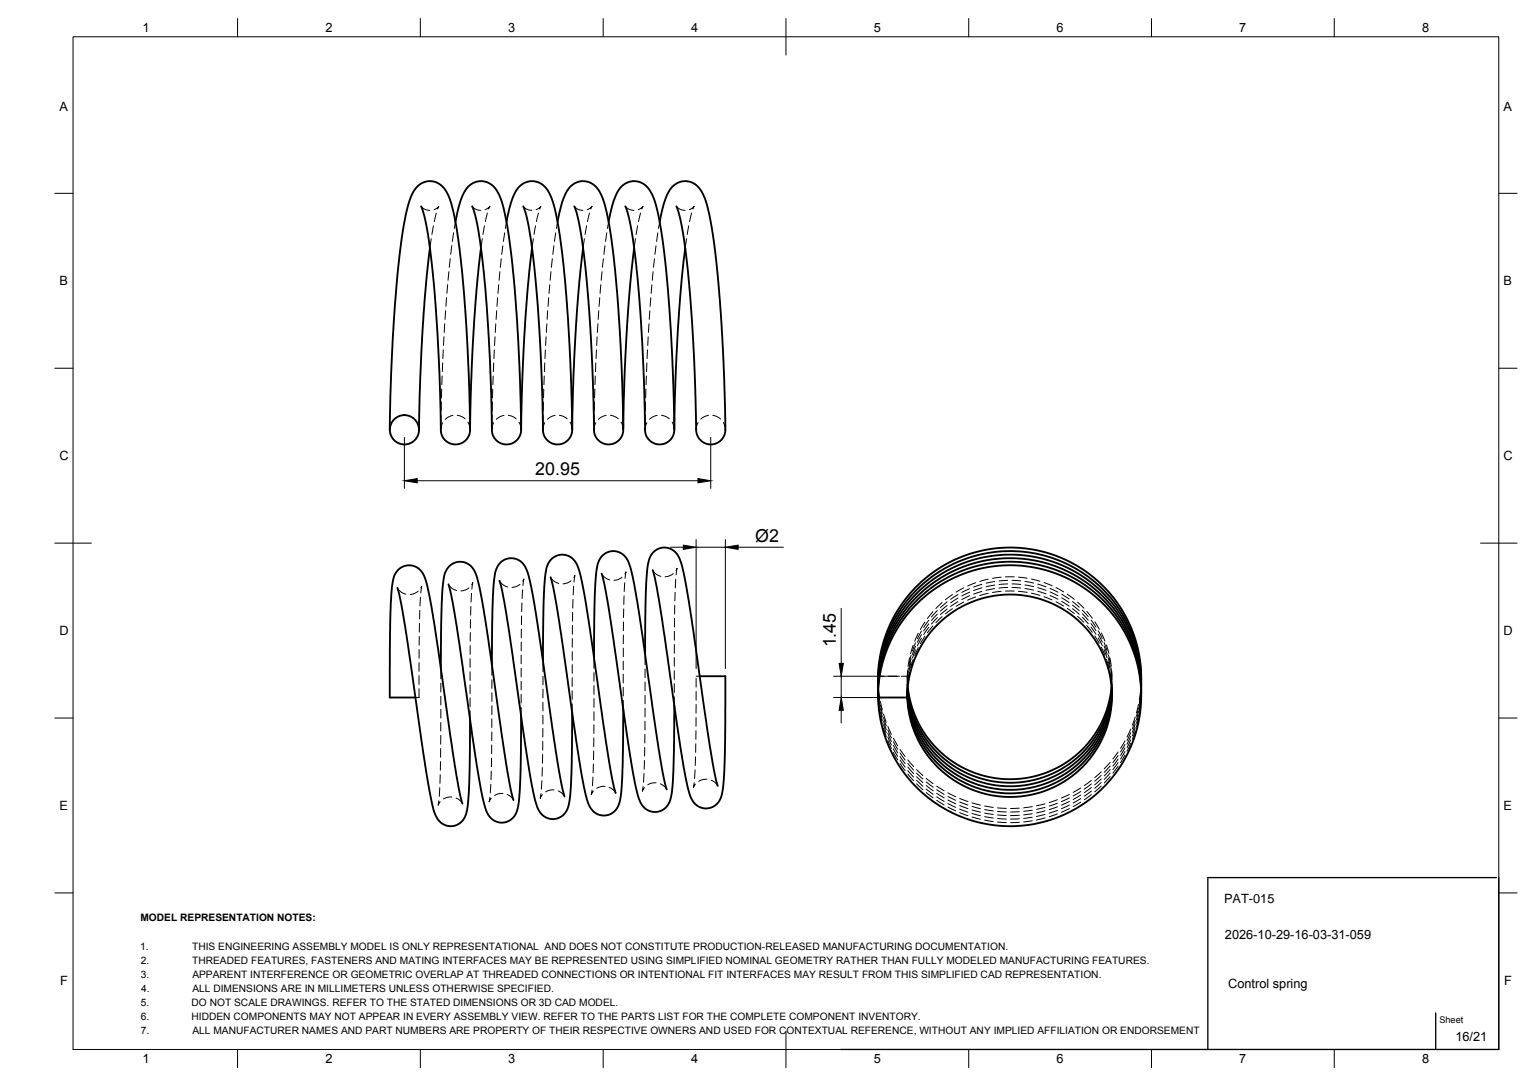
ISO-10303-21;
HEADER;
/* Generated by software containing ST-Developer
 * from STEP Tools, Inc. (www.steptools.com) 
 */

FILE_DESCRIPTION(
/* description */ ('PAT-015'),
/* implementation_level */ '2;1');

FILE_NAME(
/* name */ 'Control spring.step',
/* time_stamp */ '2026-10-29T16:03:43-07:00',
/* author */ (''),
/* organization */ (''),
/* preprocessor_version */ 'ST-DEVELOPER v20.2',
/* originating_system */ 'Autodesk Translation Framework v15.17.0.0',
/* authorisation */ '');

FILE_SCHEMA (('AUTOMOTIVE_DESIGN { 1 0 10303 214 3 1 1 }'));
ENDSEC;

DATA;
#10=MECHANICAL_DESIGN_GEOMETRIC_PRESENTATION_REPRESENTATION('',(#244),#10266);
#167=B_SPLINE_SURFACE_WITH_KNOTS('',3,3,((#8962,#8963,#8964,#8965,#8966,
#8967,#8968,#8969,#8970,#8971,#8972,#8973,#8974,#8975,#8976,#8977,#8978,
#8979,#8980,#8981,#8982,#8983,#8984,#8985,#8986,#8987,#8988,#8989,#8990,
#8991,#8992,#8993,#8994,#8995,#8996,#8997,#8998,#8999,#9000,#9001,#9002,
#9003,#9004,#9005,#9006,#9007,#9008,#9009,#9010,#9011,#9012,#9013,#9014,
#9015,#9016,#9017,#9018,#9019,#9020,#9021,#9022,#9023,#9024,#9025,#9026,
#9027,#9028,#9029,#9030,#9031,#9032),(#9033,#9034,#9035,#9036,#9037,#9038,
#9039,#9040,#9041,#9042,#9043,#9044,#9045,#9046,#9047,#9048,#9049,#9050,
#9051,#9052,#9053,#9054,#9055,#9056,#9057,#9058,#9059,#9060,#9061,#9062,
#9063,#9064,#9065,#9066,#9067,#9068,#9069,#9070,#9071,#9072,#9073,#9074,
#9075,#9076,#9077,#9078,#9079,#9080,#9081,#9082,#9083,#9084,#9085,#9086,
#9087,#9088,#9089,#9090,#9091,#9092,#9093,#9094,#9095,#9096,#9097,#9098,
#9099,#9100,#9101,#9102,#9103),(#9104,#9105,#9106,#9107,#9108,#9109,#9110,
#9111,#9112,#9113,#9114,#9115,#9116,#9117,#9118,#9119,#9120,#9121,#9122,
#9123,#9124,#9125,#9126,#9127,#9128,#9129,#9130,#9131,#9132,#9133,#9134,
#9135,#9136,#9137,#9138,#9139,#9140,#9141,#9142,#9143,#9144,#9145,#9146,
#9147,#9148,#9149,#9150,#9151,#9152,#9153,#9154,#9155,#9156,#9157,#9158,
#9159,#9160,#9161,#9162,#9163,#9164,#9165,#9166,#9167,#9168,#9169,#9170,
#9171,#9172,#9173,#9174),(#9175,#9176,#9177,#9178,#9179,#9180,#9181,#9182,
#9183,#9184,#9185,#9186,#9187,#9188,#9189,#9190,#9191,#9192,#9193,#9194,
#9195,#9196,#9197,#9198,#9199,#9200,#9201,#9202,#9203,#9204,#9205,#9206,
#9207,#9208,#9209,#9210,#9211,#9212,#9213,#9214,#9215,#9216,#9217,#9218,
#9219,#9220,#9221,#9222,#9223,#9224,#9225,#9226,#9227,#9228,#9229,#9230,
#9231,#9232,#9233,#9234,#9235,#9236,#9237,#9238,#9239,#9240,#9241,#9242,
#9243,#9244,#9245),(#9246,#9247,#9248,#9249,#9250,#9251,#9252,#9253,#9254,
#9255,#9256,#9257,#9258,#9259,#9260,#9261,#9262,#9263,#9264,#9265,#9266,
#9267,#9268,#9269,#9270,#9271,#9272,#9273,#9274,#9275,#9276,#9277,#9278,
#9279,#9280,#9281,#9282,#9283,#9284,#9285,#9286,#9287,#9288,#9289,#9290,
#9291,#9292,#9293,#9294,#9295,#9296,#9297,#9298,#9299,#9300,#9301,#9302,
#9303,#9304,#9305,#9306,#9307,#9308,#9309,#9310,#9311,#9312,#9313,#9314,
#9315,#9316),(#9317,#9318,#9319,#9320,#9321,#9322,#9323,#9324,#9325,#9326,
#9327,#9328,#9329,#9330,#9331,#9332,#9333,#9334,#9335,#9336,#9337,#9338,
#9339,#9340,#9341,#9342,#9343,#9344,#9345,#9346,#9347,#9348,#9349,#9350,
#9351,#9352,#9353,#9354,#9355,#9356,#9357,#9358,#9359,#9360,#9361,#9362,
#9363,#9364,#9365,#9366,#9367,#9368,#9369,#9370,#9371,#9372,#9373,#9374,
#9375,#9376,#9377,#9378,#9379,#9380,#9381,#9382,#9383,#9384,#9385,#9386,
#9387),(#9388,#9389,#9390,#9391,#9392,#9393,#9394,#9395,#9396,#9397,#9398,
#9399,#9400,#9401,#9402,#9403,#9404,#9405,#9406,#9407,#9408,#9409,#9410,
#9411,#9412,#9413,#9414,#9415,#9416,#9417,#9418,#9419,#9420,#9421,#9422,
#9423,#9424,#9425,#9426,#9427,#9428,#9429,#9430,#9431,#9432,#9433,#9434,
#9435,#9436,#9437,#9438,#9439,#9440,#9441,#9442,#9443,#9444,#9445,#9446,
#9447,#9448,#9449,#9450,#9451,#9452,#9453,#9454,#9455,#9456,#9457,#9458),
(#9459,#9460,#9461,#9462,#9463,#9464,#9465,#9466,#9467,#9468,#9469,#9470,
#9471,#9472,#9473,#9474,#9475,#9476,#9477,#9478,#9479,#9480,#9481,#9482,
#9483,#9484,#9485,#9486,#9487,#9488,#9489,#9490,#9491,#9492,#9493,#9494,
#9495,#9496,#9497,#9498,#9499,#9500,#9501,#9502,#9503,#9504,#9505,#9506,
#9507,#9508,#9509,#9510,#9511,#9512,#9513,#9514,#9515,#9516,#9517,#9518,
#9519,#9520,#9521,#9522,#9523,#9524,#9525,#9526,#9527,#9528,#9529),(#9530,
#9531,#9532,#9533,#9534,#9535,#9536,#9537,#9538,#9539,#9540,#9541,#9542,
#9543,#9544,#9545,#9546,#9547,#9548,#9549,#9550,#9551,#9552,#9553,#9554,
#9555,#9556,#9557,#9558,#9559,#9560,#9561,#9562,#9563,#9564,#9565,#9566,
#9567,#9568,#9569,#9570,#9571,#9572,#9573,#9574,#9575,#9576,#9577,#9578,
#9579,#9580,#9581,#9582,#9583,#9584,#9585,#9586,#9587,#9588,#9589,#9590,
#9591,#9592,#9593,#9594,#9595,#9596,#9597,#9598,#9599,#9600),(#9601,#9602,
#9603,#9604,#9605,#9606,#9607,#9608,#9609,#9610,#9611,#9612,#9613,#9614,
#9615,#9616,#9617,#9618,#9619,#9620,#9621,#9622,#9623,#9624,#9625,#9626,
#9627,#9628,#9629,#9630,#9631,#9632,#9633,#9634,#9635,#9636,#9637,#9638,
#9639,#9640,#9641,#9642,#9643,#9644,#9645,#9646,#9647,#9648,#9649,#9650,
#9651,#9652,#9653,#9654,#9655,#9656,#9657,#9658,#9659,#9660,#9661,#9662,
#9663,#9664,#9665,#9666,#9667,#9668,#9669,#9670,#9671)),.UNSPECIFIED.,.T.,
 .F.,.F.,(4,1,1,1,1,1,1,4),(4,1,1,1,1,1,1,1,1,1,1,1,1,1,1,1,1,1,1,1,1,1,
1,1,1,1,1,1,1,1,1,1,1,1,1,1,1,1,1,1,1,1,1,1,1,1,1,1,1,1,1,1,1,1,1,1,1,1,
1,1,1,1,1,1,1,1,1,1,4),(-3.14159265358979,-2.24399475256414,-1.34639685153848,
-0.448798950512828,0.448798950512828,1.34639685153848,2.24399475256414,
3.14159265358979),(0.,0.0178571428571429,0.0357142857142857,0.0535714285714286,
0.0714285714285714,0.0892857142857143,0.107142857142857,0.125,0.142857142857143,
0.150793650793651,0.158730158730159,0.174603174603175,0.19047619047619,
0.202380952380952,0.214285714285714,0.226190476190476,0.238095238095238,
0.25,0.261904761904762,0.267857142857143,0.273809523809524,0.285714285714286,
0.297619047619048,0.30952380952381,0.321428571428571,0.333333333333333,
0.349206349206349,0.365079365079365,0.380952380952381,0.396825396825397,
0.412698412698413,0.428571428571429,0.446428571428571,0.464285714285714,
0.476190476190476,0.488095238095238,0.5,0.517857142857143,0.535714285714286,
0.553571428571429,0.571428571428571,0.589285714285714,0.607142857142857,
0.625,0.642857142857143,0.660714285714286,0.678571428571428,0.696428571428571,
0.714285714285714,0.726190476190476,0.738095238095238,0.75,0.761904761904762,
0.773809523809524,0.785714285714286,0.797619047619047,0.809523809523809,
0.821428571428571,0.833333333333333,0.845238095238095,0.857142857142857,
0.875,0.892857142857143,0.910714285714286,0.928571428571429,0.946428571428571,
0.964285714285714,0.982142857142857,1.),.UNSPECIFIED.);
#196=SHAPE_REPRESENTATION_RELATIONSHIP('SRR','None',#10367,#219);
#219=ADVANCED_BREP_SHAPE_REPRESENTATION('',(#269),#10255);
#244=STYLED_ITEM('',(#10547),#269);
#269=MANIFOLD_SOLID_BREP('Body1',#4703);
#513=PLANE('',#5380);
#514=PLANE('',#5381);
#767=FACE_OUTER_BOUND('',#1164,.T.);
#768=FACE_OUTER_BOUND('',#1165,.T.);
#769=FACE_OUTER_BOUND('',#1166,.T.);
#1164=EDGE_LOOP('',(#3963,#3964,#3965,#3966));
#1165=EDGE_LOOP('',(#3967));
#1166=EDGE_LOOP('',(#3968));
#1319=B_SPLINE_CURVE_WITH_KNOTS('',3,(#9675,#9676,#9677,#9678,#9679,#9680,
#9681,#9682,#9683,#9684,#9685,#9686,#9687,#9688,#9689,#9690,#9691,#9692,
#9693,#9694,#9695,#9696,#9697,#9698,#9699,#9700,#9701,#9702,#9703,#9704,
#9705,#9706,#9707,#9708,#9709,#9710,#9711,#9712,#9713,#9714,#9715,#9716,
#9717,#9718,#9719,#9720,#9721,#9722,#9723,#9724,#9725,#9726,#9727,#9728,
#9729,#9730,#9731,#9732,#9733,#9734,#9735,#9736,#9737,#9738,#9739,#9740,
#9741,#9742,#9743,#9744,#9745),.UNSPECIFIED.,.F.,.F.,(4,1,1,1,1,1,1,1,1,
1,1,1,1,1,1,1,1,1,1,1,1,1,1,1,1,1,1,1,1,1,1,1,1,1,1,1,1,1,1,1,1,1,1,1,1,
1,1,1,1,1,1,1,1,1,1,1,1,1,1,1,1,1,1,1,1,1,1,1,4),(0.,0.0178571428571429,
0.0357142857142857,0.0535714285714286,0.0714285714285714,0.0892857142857143,
0.107142857142857,0.125,0.142857142857143,0.150793650793651,0.158730158730159,
0.174603174603175,0.19047619047619,0.202380952380952,0.214285714285714,
0.226190476190476,0.238095238095238,0.25,0.261904761904762,0.267857142857143,
0.273809523809524,0.285714285714286,0.297619047619048,0.30952380952381,
0.321428571428571,0.333333333333333,0.349206349206349,0.365079365079365,
0.380952380952381,0.396825396825397,0.412698412698413,0.428571428571429,
0.446428571428571,0.464285714285714,0.476190476190476,0.488095238095238,
0.5,0.517857142857143,0.535714285714286,0.553571428571429,0.571428571428571,
0.589285714285714,0.607142857142857,0.625,0.642857142857143,0.660714285714286,
0.678571428571428,0.696428571428571,0.714285714285714,0.726190476190476,
0.738095238095238,0.75,0.761904761904762,0.773809523809524,0.785714285714286,
0.797619047619047,0.809523809523809,0.821428571428571,0.833333333333333,
0.845238095238095,0.857142857142857,0.875,0.892857142857143,0.910714285714286,
0.928571428571429,0.946428571428571,0.964285714285714,0.982142857142857,
1.),.UNSPECIFIED.);
#2067=CIRCLE('',#5378,0.1);
#2068=CIRCLE('',#5379,0.1);
#2401=VERTEX_POINT('',#9672);
#2402=VERTEX_POINT('',#9674);
#2937=EDGE_CURVE('',#2401,#2401,#2067,.T.);
#2938=EDGE_CURVE('',#2401,#2402,#1319,.T.);
#2939=EDGE_CURVE('',#2402,#2402,#2068,.T.);
#3963=ORIENTED_EDGE('',*,*,#2937,.T.);
#3964=ORIENTED_EDGE('',*,*,#2938,.T.);
#3965=ORIENTED_EDGE('',*,*,#2939,.F.);
#3966=ORIENTED_EDGE('',*,*,#2938,.F.);
#3967=ORIENTED_EDGE('',*,*,#2939,.T.);
#3968=ORIENTED_EDGE('',*,*,#2937,.F.);
#4602=ADVANCED_FACE('',(#767),#167,.T.);
#4603=ADVANCED_FACE('',(#768),#513,.T.);
#4604=ADVANCED_FACE('',(#769),#514,.F.);
#4703=CLOSED_SHELL('',(#4602,#4603,#4604));
#5377=AXIS2_PLACEMENT_3D('',#8961,#6549,#6550);
#5378=AXIS2_PLACEMENT_3D('',#9673,#6551,#6552);
#5379=AXIS2_PLACEMENT_3D('',#9746,#6553,#6554);
#5380=AXIS2_PLACEMENT_3D('',#9747,#6555,#6556);
#5381=AXIS2_PLACEMENT_3D('',#9748,#6557,#6558);
#6549=DIRECTION('axis',(0.,0.,1.));
#6550=DIRECTION('refdir',(1.,0.,0.));
#6551=DIRECTION('center_axis',(-0.000134591856444243,0.997598919682403,
0.0692558830247305));
#6552=DIRECTION('ref_axis',(9.34371278597603E-6,-0.0692558823944232,0.997598928761687));
#6553=DIRECTION('center_axis',(0.000134591670588553,0.997598919668532,0.0692558832248945));
#6554=DIRECTION('ref_axis',(-0.499431472094232,0.0600671278230296,-0.864268560597272));
#6555=DIRECTION('center_axis',(0.000134591670588553,0.997598919668532,0.0692558832248945));
#6556=DIRECTION('ref_axis',(-0.499431472094232,0.0600671278230296,-0.864268560597272));
#6557=DIRECTION('center_axis',(-0.000134591856444243,0.997598919682403,
0.0692558830247305));
#6558=DIRECTION('ref_axis',(9.34371278597603E-6,-0.0692558823944232,0.997598928761687));
#8961=CARTESIAN_POINT('',(0.,0.,0.));
#8962=CARTESIAN_POINT('Ctrl Pts',(0.799999065628721,0.00692558823944229,
5.30024010712383));
#8963=CARTESIAN_POINT('Ctrl Pts',(0.799974755250737,0.187114846749742,5.31274930893178));
#8964=CARTESIAN_POINT('Ctrl Pts',(0.674578200671659,0.546127076651831,5.33781512365923));
#8965=CARTESIAN_POINT('Ctrl Pts',(0.187998995393781,0.852903359039399,5.37564381521248));
#8966=CARTESIAN_POINT('Ctrl Pts',(-0.386721866921525,0.788448388841122,
5.41368605209984));
#8967=CARTESIAN_POINT('Ctrl Pts',(-0.7983994419892,0.377627224111744,5.45194644400096));
#8968=CARTESIAN_POINT('Ctrl Pts',(-0.864375113399524,-0.203617876612744,
5.49042055747836));
#8969=CARTESIAN_POINT('Ctrl Pts',(-0.552019639313923,-0.701812288635587,
5.52910737914477));
#8970=CARTESIAN_POINT('Ctrl Pts',(0.00615426428515267,-0.897757418326962,
5.56800374230524));
#8971=CARTESIAN_POINT('Ctrl Pts',(0.463089276607972,-0.737891299975203,
5.59986549204054));
#8972=CARTESIAN_POINT('Ctrl Pts',(0.706662565433678,-0.474149107376678,
5.62457829573124));
#8973=CARTESIAN_POINT('Ctrl Pts',(0.854347338563578,-0.169471123140589,
5.6478904398873));
#8974=CARTESIAN_POINT('Ctrl Pts',(0.854381411403854,0.269671075667267,5.67712918390586));
#8975=CARTESIAN_POINT('Ctrl Pts',(0.581578462406747,0.670744438556907,5.70943359497258));
#8976=CARTESIAN_POINT('Ctrl Pts',(0.189982000930166,0.858805851522918,5.73891161848027));
#8977=CARTESIAN_POINT('Ctrl Pts',(-0.201854620920769,0.859148371452269,
5.76552549972421));
#8978=CARTESIAN_POINT('Ctrl Pts',(-0.556170302204947,0.688486751453872,
5.79222147180784));
#8979=CARTESIAN_POINT('Ctrl Pts',(-0.802120584542054,0.380288702719923,
5.81899788702529));
#8980=CARTESIAN_POINT('Ctrl Pts',(-0.890321102734134,-0.0053444036833259,
5.84585301727138));
#8981=CARTESIAN_POINT('Ctrl Pts',(-0.816781798992104,-0.327577127496462,
5.86829638740099));
#8982=CARTESIAN_POINT('Ctrl Pts',(-0.678277859648778,-0.547664335405585,
5.88628859994389));
#8983=CARTESIAN_POINT('Ctrl Pts',(-0.494316135451619,-0.731945478665225,
5.90430550175064));
#8984=CARTESIAN_POINT('Ctrl Pts',(-0.194941007989142,-0.876310026230692,
5.92687230420244));
#8985=CARTESIAN_POINT('Ctrl Pts',(0.204945568353256,-0.876409485122255,
5.95402353339188));
#8986=CARTESIAN_POINT('Ctrl Pts',(0.566325487118899,-0.702556101088839,
5.98124373289334));
#8987=CARTESIAN_POINT('Ctrl Pts',(0.816751045229916,-0.388463305588866,
6.00853075028047));
#8988=CARTESIAN_POINT('Ctrl Pts',(0.917174982875959,0.0480250206861584,
6.03892142694837));
#8989=CARTESIAN_POINT('Ctrl Pts',(0.768829350780382,0.528866010776267,6.07244001895545));
#8990=CARTESIAN_POINT('Ctrl Pts',(0.338627495917749,0.872873034891815,6.10911095186911));
#8991=CARTESIAN_POINT('Ctrl Pts',(-0.212178222814091,0.914151313349766,
6.14588130840082));
#8992=CARTESIAN_POINT('Ctrl Pts',(-0.691759933067223,0.637451614256161,
6.18274515756461));
#8993=CARTESIAN_POINT('Ctrl Pts',(-0.932934482256533,0.137697594997002,
6.21969639210087));
#8994=CARTESIAN_POINT('Ctrl Pts',(-0.84730393945114,-0.435496308403701,
6.25827178793966));
#8995=CARTESIAN_POINT('Ctrl Pts',(-0.415273257958933,-0.868240176171726,
6.29847623644814));
#8996=CARTESIAN_POINT('Ctrl Pts',(0.146189896678077,-0.930950222024402,
6.33566388079779));
#8997=CARTESIAN_POINT('Ctrl Pts',(0.578787425776111,-0.722091726547751,
6.36825221458814));
#8998=CARTESIAN_POINT('Ctrl Pts',(0.835229259505866,-0.400278931762148,
6.3962159259868));
#8999=CARTESIAN_POINT('Ctrl Pts',(0.943177486850013,0.0688606453452641,
6.42887288667825));
#9000=CARTESIAN_POINT('Ctrl Pts',(0.756462512495389,0.604750444420971,6.46623690685835));
#9001=CARTESIAN_POINT('Ctrl Pts',(0.214509054547464,0.945343920852135,6.50831791566041));
#9002=CARTESIAN_POINT('Ctrl Pts',(-0.421585054233784,0.873670673138226,
6.55043539297339));
#9003=CARTESIAN_POINT('Ctrl Pts',(-0.874725713994987,0.420703846750279,
6.59257924943873));
#9004=CARTESIAN_POINT('Ctrl Pts',(-0.946491736933492,-0.216206220818672,
6.63473932973225));
#9005=CARTESIAN_POINT('Ctrl Pts',(-0.605472064685913,-0.758979181442101,
6.67690544450194));
#9006=CARTESIAN_POINT('Ctrl Pts',(-0.000509641250504898,-0.970641038681315,
6.71906739492544));
#9007=CARTESIAN_POINT('Ctrl Pts',(0.604236817182525,-0.758999928674301,
6.76121498571335));
#9008=CARTESIAN_POINT('Ctrl Pts',(0.944676427167983,-0.216670516455945,
6.80333805746961));
#9009=CARTESIAN_POINT('Ctrl Pts',(0.873719648783539,0.418956634979468,6.8454265042638));
#9010=CARTESIAN_POINT('Ctrl Pts',(0.421037273012308,0.871132652579719,6.88747029453994));
#9011=CARTESIAN_POINT('Ctrl Pts',(-0.142342851291253,0.933831870869633,
6.92479402146672));
#9012=CARTESIAN_POINT('Ctrl Pts',(-0.575104466317865,0.724476767443434,
6.95741054274359));
#9013=CARTESIAN_POINT('Ctrl Pts',(-0.831597121038275,0.403171008458228,
6.98533606563364));
#9014=CARTESIAN_POINT('Ctrl Pts',(-0.922808904665035,0.00254068286457492,
7.01322724854536));
#9015=CARTESIAN_POINT('Ctrl Pts',(-0.831484359832733,-0.397369041930912,
7.04108128388358));
#9016=CARTESIAN_POINT('Ctrl Pts',(-0.576024516479058,-0.717622866946566,
7.06889539860548));
#9017=CARTESIAN_POINT('Ctrl Pts',(-0.207464718971416,-0.895095126308869,
7.09666685370961));
#9018=CARTESIAN_POINT('Ctrl Pts',(0.200869050822812,-0.894893573965507,
7.12439296344474));
#9019=CARTESIAN_POINT('Ctrl Pts',(0.568135301656786,-0.717941543510051,
7.15207107099507));
#9020=CARTESIAN_POINT('Ctrl Pts',(0.821742493579341,-0.399813712939291,
7.17969857736332));
#9021=CARTESIAN_POINT('Ctrl Pts',(0.912100647381109,-0.00372699171446918,
7.20727292857109));
#9022=CARTESIAN_POINT('Ctrl Pts',(0.821667160899362,0.391120281113409,7.23479162069698));
#9023=CARTESIAN_POINT('Ctrl Pts',(0.527798142032111,0.760706416566583,7.26682897888736));
#9024=CARTESIAN_POINT('Ctrl Pts',(0.00437094025093319,0.944184514671381,
7.30334225024583));
#9025=CARTESIAN_POINT('Ctrl Pts',(-0.583164611559206,0.738086874931468,
7.3442757526392));
#9026=CARTESIAN_POINT('Ctrl Pts',(-0.912546668924433,0.213026529714121,
7.38505770065783));
#9027=CARTESIAN_POINT('Ctrl Pts',(-0.843060529623956,-0.400706652853849,
7.42568118182012));
#9028=CARTESIAN_POINT('Ctrl Pts',(-0.407835437985135,-0.835237258109269,
7.46613873367218));
#9029=CARTESIAN_POINT('Ctrl Pts',(0.200737244244076,-0.903598468057941,
7.5064251969444));
#9030=CARTESIAN_POINT('Ctrl Pts',(0.71672352100227,-0.578479045751934,7.54653146106904));
#9031=CARTESIAN_POINT('Ctrl Pts',(0.849917343436364,-0.197265324952655,
7.57314919120958));
#9032=CARTESIAN_POINT('Ctrl Pts',(0.849943147209423,-0.00600671278230411,
7.58642685605973));
#9033=CARTESIAN_POINT('Ctrl Pts',(0.770079135866838,0.00692155156817904,
5.30024010712383));
#9034=CARTESIAN_POINT('Ctrl Pts',(0.770055720112496,0.180479832525886,5.31228896941391));
#9035=CARTESIAN_POINT('Ctrl Pts',(0.649347137055222,0.526118956744516,5.33641790275693));
#9036=CARTESIAN_POINT('Ctrl Pts',(0.180677599950648,0.821679099419469,5.37285586761231));
#9037=CARTESIAN_POINT('Ctrl Pts',(-0.373128354027995,0.759596327571503,
5.40950951731212));
#9038=CARTESIAN_POINT('Ctrl Pts',(-0.770051450984494,0.363580245990391,
5.44639246645647));
#9039=CARTESIAN_POINT('Ctrl Pts',(-0.833750732775199,-0.197081341774288,
5.48350071817735));
#9040=CARTESIAN_POINT('Ctrl Pts',(-0.532331315046715,-0.677969641751496,
5.5208364575171));
#9041=CARTESIAN_POINT('Ctrl Pts',(0.00675318837749655,-0.867294541965757,
5.558400781988));
#9042=CARTESIAN_POINT('Ctrl Pts',(0.448424688054875,-0.712845112569316,
5.58919119813692));
#9043=CARTESIAN_POINT('Ctrl Pts',(0.684012778929899,-0.457765801730765,
5.61309167265538));
#9044=CARTESIAN_POINT('Ctrl Pts',(0.82691455168644,-0.162993811747473,5.6356443242608));
#9045=CARTESIAN_POINT('Ctrl Pts',(0.82699649983482,0.262124971545771,5.66394696022895));
#9046=CARTESIAN_POINT('Ctrl Pts',(0.562750276158912,0.650752034831193,5.69524212629919));
#9047=CARTESIAN_POINT('Ctrl Pts',(0.183080725565527,0.833119661747386,5.72381920452852));
#9048=CARTESIAN_POINT('Ctrl Pts',(-0.197084703463694,0.833490239824234,
5.74963623066415));
#9049=CARTESIAN_POINT('Ctrl Pts',(-0.541119975074503,0.667809968168665,
5.77555492059187));
#9050=CARTESIAN_POINT('Ctrl Pts',(-0.780113947482257,0.368392103745768,
5.80156649252668));
#9051=CARTESIAN_POINT('Ctrl Pts',(-0.865905134963049,-0.00656170868815412,
5.82767483842523));
#9052=CARTESIAN_POINT('Ctrl Pts',(-0.794375852743549,-0.320111204417347,
5.84950881094256));
#9053=CARTESIAN_POINT('Ctrl Pts',(-0.659521269028743,-0.534410811061921,
5.86702622272765));
#9054=CARTESIAN_POINT('Ctrl Pts',(-0.480335340635082,-0.713917263728105,
5.88457460840773));
#9055=CARTESIAN_POINT('Ctrl Pts',(-0.188587087034294,-0.854642083096481,
5.90656315000717));
#9056=CARTESIAN_POINT('Ctrl Pts',(0.201462529249485,-0.854779640403169,
5.9330427097564));
#9057=CARTESIAN_POINT('Ctrl Pts',(0.554262072476138,-0.685098200004362,
5.95961046024728));
#9058=CARTESIAN_POINT('Ctrl Pts',(0.798967352085236,-0.378235706832728,
5.98626742358202));
#9059=CARTESIAN_POINT('Ctrl Pts',(0.89721847916451,0.0485845903033819,6.01597993297972));
#9060=CARTESIAN_POINT('Ctrl Pts',(0.752070839701578,0.519313731169816,6.04878757680353));
#9061=CARTESIAN_POINT('Ctrl Pts',(0.330497979661169,0.856564661134425,6.08472490306161));
#9062=CARTESIAN_POINT('Ctrl Pts',(-0.209973066601811,0.897165035883339,
6.12079612560753));
#9063=CARTESIAN_POINT('Ctrl Pts',(-0.68120970786282,0.625397209779933,6.15700765884533));
#9064=CARTESIAN_POINT('Ctrl Pts',(-0.918572438612158,0.13378828614086,6.19335554838198));
#9065=CARTESIAN_POINT('Ctrl Pts',(-0.83433799028855,-0.430850802296383,
6.23134861625561));
#9066=CARTESIAN_POINT('Ctrl Pts',(-0.408316865658928,-0.857793214073537,
6.2709938323838));
#9067=CARTESIAN_POINT('Ctrl Pts',(0.146288162282126,-0.919868958459814,
6.30771962173879));
#9068=CARTESIAN_POINT('Ctrl Pts',(0.574223288772557,-0.71333190916663,6.33995134748923));
#9069=CARTESIAN_POINT('Ctrl Pts',(0.828161465810104,-0.394717048019018,
6.36763553346922));
#9070=CARTESIAN_POINT('Ctrl Pts',(0.935214831817973,0.0702367246280078,
6.39999872706231));
#9071=CARTESIAN_POINT('Ctrl Pts',(0.750063250540666,0.602049612066996,6.43706602732403));
#9072=CARTESIAN_POINT('Ctrl Pts',(0.211520380136952,0.940697836629915,6.47888152979277));
#9073=CARTESIAN_POINT('Ctrl Pts',(-0.421676436247289,0.869510362169926,
6.52079671898647));
#9074=CARTESIAN_POINT('Ctrl Pts',(-0.873553921061096,0.418039168812721,
6.56280406058959));
#9075=CARTESIAN_POINT('Ctrl Pts',(-0.945379508760524,-0.217899113421901,
6.60489250808515));
#9076=CARTESIAN_POINT('Ctrl Pts',(-0.604485708962148,-0.760787236561161,
6.64705240063428));
#9077=CARTESIAN_POINT('Ctrl Pts',(0.00138176225817566,-0.972945250150102,
6.6892731978663));
#9078=CARTESIAN_POINT('Ctrl Pts',(0.608080140735397,-0.760798630125154,
6.73154461863783));
#9079=CARTESIAN_POINT('Ctrl Pts',(0.950239792824421,-0.216025881173973,
6.77385551750453));
#9080=CARTESIAN_POINT('Ctrl Pts',(0.879017289772042,0.423590907490335,6.81620268596198));
#9081=CARTESIAN_POINT('Ctrl Pts',(0.422960901581898,0.879362908068112,6.85856017311708));
#9082=CARTESIAN_POINT('Ctrl Pts',(-0.145593093231334,0.942790559668914,
6.89621968364161));
#9083=CARTESIAN_POINT('Ctrl Pts',(-0.582932490358213,0.73127758858104,6.92917512678282));
#9084=CARTESIAN_POINT('Ctrl Pts',(-0.842401988544835,0.406320842666593,
6.957415448388));
#9085=CARTESIAN_POINT('Ctrl Pts',(-0.934795701286156,0.000685604828614038,
6.985653769321));
#9086=CARTESIAN_POINT('Ctrl Pts',(-0.842294766840471,-0.404603381671274,
7.01387715318084));
#9087=CARTESIAN_POINT('Ctrl Pts',(-0.583187447906784,-0.729494778082508,
7.04208836805485));
#9088=CARTESIAN_POINT('Ctrl Pts',(-0.20899792340701,-0.909726737101999,
7.07028057033796));
#9089=CARTESIAN_POINT('Ctrl Pts',(0.206012719667752,-0.909558569724805,
7.09845804612497));
#9090=CARTESIAN_POINT('Ctrl Pts',(0.579624839727756,-0.72959465407811,7.12660922044297));
#9091=CARTESIAN_POINT('Ctrl Pts',(0.837867106227739,-0.405711083857505,
7.15473493621397));
#9092=CARTESIAN_POINT('Ctrl Pts',(0.929983985732294,-0.00207542308664412,
7.18283200361311));
#9093=CARTESIAN_POINT('Ctrl Pts',(0.837775922394786,0.40066931879227,7.21089711007051));
#9094=CARTESIAN_POINT('Ctrl Pts',(0.537807840870324,0.777996358577212,7.24360025784798));
#9095=CARTESIAN_POINT('Ctrl Pts',(0.00294143852372089,0.965597941956312,
7.28090792189502));
#9096=CARTESIAN_POINT('Ctrl Pts',(-0.59827790503141,0.754837569025208,7.32278668150169));
#9097=CARTESIAN_POINT('Ctrl Pts',(-0.935814946990508,0.217001877726337,
7.36456027598379));
#9098=CARTESIAN_POINT('Ctrl Pts',(-0.864667175323564,-0.412475523451113,
7.40622093849563));
#9099=CARTESIAN_POINT('Ctrl Pts',(-0.417866766747618,-0.858729006758795,
7.44775776125507));
#9100=CARTESIAN_POINT('Ctrl Pts',(0.207655975088153,-0.929085997388315,
7.48916462895728));
#9101=CARTESIAN_POINT('Ctrl Pts',(0.73862266392267,-0.594662305466805,7.53042707168622));
#9102=CARTESIAN_POINT('Ctrl Pts',(0.875837799539084,-0.201989676969171,
7.55784229424685));
#9103=CARTESIAN_POINT('Ctrl Pts',(0.875864379853922,-0.00497530564290791,
7.5715195387037));
#9104=CARTESIAN_POINT('Ctrl Pts',(0.710428941733949,0.00492953088558486,
5.32881831830437));
#9105=CARTESIAN_POINT('Ctrl Pts',(0.71040731614315,0.165219065394011,5.33994603008611));
#9106=CARTESIAN_POINT('Ctrl Pts',(0.599024128589712,0.483870366740507,5.3621924509196));
#9107=CARTESIAN_POINT('Ctrl Pts',(0.167205166996449,0.75612127364975,5.39576440291455));
#9108=CARTESIAN_POINT('Ctrl Pts',(-0.342469011252512,0.698867316238289,
5.42949607339388));
#9109=CARTESIAN_POINT('Ctrl Pts',(-0.707447256311363,0.334638873927445,
5.46341601587375));
#9110=CARTESIAN_POINT('Ctrl Pts',(-0.765942731942805,-0.180685845273631,
5.49752276624412));
#9111=CARTESIAN_POINT('Ctrl Pts',(-0.488977975671522,-0.622493468082251,
5.53182729600019));
#9112=CARTESIAN_POINT('Ctrl Pts',(0.00623870066985125,-0.79639957834953,
5.56633555615365));
#9113=CARTESIAN_POINT('Ctrl Pts',(0.411979748797062,-0.65451285296037,5.59462344155862));
#9114=CARTESIAN_POINT('Ctrl Pts',(0.628431910779513,-0.420156210117234,
5.61658281146561));
#9115=CARTESIAN_POINT('Ctrl Pts',(0.759739764112401,-0.149292484888909,
5.63730747934422));
#9116=CARTESIAN_POINT('Ctrl Pts',(0.759837930575591,0.241447639232068,5.66332246132793));
#9117=CARTESIAN_POINT('Ctrl Pts',(0.516864570620339,0.598828714990839,5.6921027083035));
#9118=CARTESIAN_POINT('Ctrl Pts',(0.16754402090728,0.766642660816134,5.7183984452765));
#9119=CARTESIAN_POINT('Ctrl Pts',(-0.18243289406626,0.766996703299491,5.74216819224318));
#9120=CARTESIAN_POINT('Ctrl Pts',(-0.499344694617947,0.614409373974203,
5.7660436717059));
#9121=CARTESIAN_POINT('Ctrl Pts',(-0.719666388043044,0.338417073722969,
5.79002421526266));
#9122=CARTESIAN_POINT('Ctrl Pts',(-0.798838486989696,-0.00747184320142611,
5.81411179267834));
#9123=CARTESIAN_POINT('Ctrl Pts',(-0.732821087254027,-0.296979929993814,
5.83427424859502));
#9124=CARTESIAN_POINT('Ctrl Pts',(-0.608236501384017,-0.494969333219339,
5.85045910955365));
#9125=CARTESIAN_POINT('Ctrl Pts',(-0.442617486739659,-0.660891288693568,
5.8666802534398));
#9126=CARTESIAN_POINT('Ctrl Pts',(-0.172748327050428,-0.791093551297648,
5.88702427548063));
#9127=CARTESIAN_POINT('Ctrl Pts',(0.188434824933959,-0.791259517626132,
5.91154722254856));
#9128=CARTESIAN_POINT('Ctrl Pts',(0.515509148139609,-0.63399975107043,5.93618028019028));
#9129=CARTESIAN_POINT('Ctrl Pts',(0.742660619778638,-0.349226128508519,
5.96092404661359));
#9130=CARTESIAN_POINT('Ctrl Pts',(0.834013573979388,0.047387173011833,5.98854018010049));
#9131=CARTESIAN_POINT('Ctrl Pts',(0.699054298781812,0.485509196729349,6.01907630606175));
#9132=CARTESIAN_POINT('Ctrl Pts',(0.306089489608805,0.800037047528466,6.05258598067156));
#9133=CARTESIAN_POINT('Ctrl Pts',(-0.198806257075136,0.83811783046203,6.08629244673437));
#9134=CARTESIAN_POINT('Ctrl Pts',(-0.639994604888811,0.58386009688861,6.12019546148202));
#9135=CARTESIAN_POINT('Ctrl Pts',(-0.862778510831916,0.122809110352501,
6.15429381358228));
#9136=CARTESIAN_POINT('Ctrl Pts',(-0.783768475044449,-0.408002461396071,
6.19001514975991));
#9137=CARTESIAN_POINT('Ctrl Pts',(-0.382461984654271,-0.810530499122485,
6.22738726758261));
#9138=CARTESIAN_POINT('Ctrl Pts',(0.141571880318707,-0.869426431241229,
6.26209856247513));
#9139=CARTESIAN_POINT('Ctrl Pts',(0.546857792365987,-0.673923824775829,
6.29262411862805));
#9140=CARTESIAN_POINT('Ctrl Pts',(0.787850231799947,-0.371686474029746,
6.31889326617887));
#9141=CARTESIAN_POINT('Ctrl Pts',(0.889701212277186,0.0702541647771362,
6.34966096595927));
#9142=CARTESIAN_POINT('Ctrl Pts',(0.713512875154728,0.577124702757749,6.38499463961466));
#9143=CARTESIAN_POINT('Ctrl Pts',(0.198967909509621,0.901053551471294,6.42496855240101));
#9144=CARTESIAN_POINT('Ctrl Pts',(-0.408089575093021,0.833131022176632,
6.46516128973043));
#9145=CARTESIAN_POINT('Ctrl Pts',(-0.842862380754781,0.399211540997894,
6.50556671739343));
#9146=CARTESIAN_POINT('Ctrl Pts',(-0.912482057616401,-0.214227019813974,
6.54617863195434));
#9147=CARTESIAN_POINT('Ctrl Pts',(-0.582857572239619,-0.739804921207224,
6.58699019870486));
#9148=CARTESIAN_POINT('Ctrl Pts',(0.00529210032697009,-0.946120388887076,
6.62799422182894));
#9149=CARTESIAN_POINT('Ctrl Pts',(0.596417413889089,-0.73978975515068,6.66918308377763));
#9150=CARTESIAN_POINT('Ctrl Pts',(0.931157121946736,-0.20751322428765,6.71054882574604));
#9151=CARTESIAN_POINT('Ctrl Pts',(0.861650483779265,0.419727599707763,6.75208097200662));
#9152=CARTESIAN_POINT('Ctrl Pts',(0.413147604956643,0.868498049400113,6.79377525221771));
#9153=CARTESIAN_POINT('Ctrl Pts',(-0.148210983168275,0.931421962876526,
6.83097036528324));
#9154=CARTESIAN_POINT('Ctrl Pts',(-0.581294729795694,0.722118347875597,
6.86360544825447));
#9155=CARTESIAN_POINT('Ctrl Pts',(-0.838871906802363,0.399682199015836,
6.89163933377065));
#9156=CARTESIAN_POINT('Ctrl Pts',(-0.930877231252504,-0.00373870819751691,
6.91972773631357));
#9157=CARTESIAN_POINT('Ctrl Pts',(-0.838749751075799,-0.407817095097561,
6.94787183402895));
#9158=CARTESIAN_POINT('Ctrl Pts',(-0.579931993725618,-0.732521582072749,
6.9760659349542));
#9159=CARTESIAN_POINT('Ctrl Pts',(-0.205212822112969,-0.913124822787424,
7.00430873475179));
#9160=CARTESIAN_POINT('Ctrl Pts',(0.211338054228992,-0.913070414334495,
7.03259350527625));
#9161=CARTESIAN_POINT('Ctrl Pts',(0.587263134138024,-0.732110657981568,
7.06092123472863));
#9162=CARTESIAN_POINT('Ctrl Pts',(0.847742099102453,-0.405599817717801,
7.08928670598057));
#9163=CARTESIAN_POINT('Ctrl Pts',(0.940948978785284,0.00228770078596691,
7.1176867396323));
#9164=CARTESIAN_POINT('Ctrl Pts',(0.847659354457111,0.410238520315532,7.14611819660086));
#9165=CARTESIAN_POINT('Ctrl Pts',(0.543275903219406,0.793339172582683,7.17932027275837));
#9166=CARTESIAN_POINT('Ctrl Pts',(-0.001093578869141,0.984623315384901,
7.21730924712761));
#9167=CARTESIAN_POINT('Ctrl Pts',(-0.615252284949225,0.769726133995085,
7.26008973650359));
#9168=CARTESIAN_POINT('Ctrl Pts',(-0.961422256849412,0.218820343216691,
7.30290266259028));
#9169=CARTESIAN_POINT('Ctrl Pts',(-0.888633848724617,-0.428292780832149,
7.34573759998394));
#9170=CARTESIAN_POINT('Ctrl Pts',(-0.42811642962634,-0.888746898872104,
7.38857936211361));
#9171=CARTESIAN_POINT('Ctrl Pts',(0.218959376739582,-0.961833511797225,
7.43142516328682));
#9172=CARTESIAN_POINT('Ctrl Pts',(0.770122900311167,-0.615157339727794,
7.47424382285298));
#9173=CARTESIAN_POINT('Ctrl Pts',(0.913207865694905,-0.206388594750497,
7.5027957331042));
#9174=CARTESIAN_POINT('Ctrl Pts',(0.913235549072487,-0.00119827763899913,
7.51704057274925));
#9175=CARTESIAN_POINT('Ctrl Pts',(0.688502394196997,-0.00177585944161231,
5.42536374837757));
#9176=CARTESIAN_POINT('Ctrl Pts',(0.688481448875166,0.153471500858794,5.43614141945633));
#9177=CARTESIAN_POINT('Ctrl Pts',(0.580508040541705,0.46124670025465,5.45764245524231));
#9178=CARTESIAN_POINT('Ctrl Pts',(0.165662319023174,0.722161337503787,5.48987538957648));
#9179=CARTESIAN_POINT('Ctrl Pts',(-0.320578571387279,0.667050889553626,
5.52206618528612));
#9180=CARTESIAN_POINT('Ctrl Pts',(-0.666378826232044,0.32127882597957,5.55424091986707));
#9181=CARTESIAN_POINT('Ctrl Pts',(-0.721063694800031,-0.164642450695304,
5.58640440743116));
#9182=CARTESIAN_POINT('Ctrl Pts',(-0.461013415699651,-0.578597703078686,
5.61857188153771));
#9183=CARTESIAN_POINT('Ctrl Pts',(0.000868763121645957,-0.740322038056404,
5.65075229330461));
#9184=CARTESIAN_POINT('Ctrl Pts',(0.377087016267437,-0.608394442936668,
5.67699673395361));
#9185=CARTESIAN_POINT('Ctrl Pts',(0.577057627822796,-0.391810817241549,
5.69729012722977));
#9186=CARTESIAN_POINT('Ctrl Pts',(0.698092236754842,-0.142020837867168,
5.71640197572506));
#9187=CARTESIAN_POINT('Ctrl Pts',(0.697963439505406,0.21710900600399,5.74031529151263));
#9188=CARTESIAN_POINT('Ctrl Pts',(0.475355133020151,0.544099194249106,5.76666169992576));
#9189=CARTESIAN_POINT('Ctrl Pts',(0.156654851678278,0.697080460332168,5.79065302227195));
#9190=CARTESIAN_POINT('Ctrl Pts',(-0.161711917448867,0.697304453295988,
5.81227877536069));
#9191=CARTESIAN_POINT('Ctrl Pts',(-0.449161842092396,0.558802207686871,
5.83393922469739));
#9192=CARTESIAN_POINT('Ctrl Pts',(-0.648454473279016,0.309008113535057,
5.85564132087709));
#9193=CARTESIAN_POINT('Ctrl Pts',(-0.719837707005216,-0.00322310267600228,
5.8773860839056));
#9194=CARTESIAN_POINT('Ctrl Pts',(-0.660324209075774,-0.263926195140504,
5.89554604949557));
#9195=CARTESIAN_POINT('Ctrl Pts',(-0.548312630732919,-0.441913047209008,
5.91009721234879));
#9196=CARTESIAN_POINT('Ctrl Pts',(-0.399568209162923,-0.590912445741052,
5.92466534563453));
#9197=CARTESIAN_POINT('Ctrl Pts',(-0.157550820881924,-0.70761172499092,
5.94291010238594));
#9198=CARTESIAN_POINT('Ctrl Pts',(0.165683821816319,-0.707692893763189,
5.96485832442363));
#9199=CARTESIAN_POINT('Ctrl Pts',(0.457834734757014,-0.567156151977817,
5.98686542599537));
#9200=CARTESIAN_POINT('Ctrl Pts',(0.660365135739603,-0.313163685177989,
6.00893343132688));
#9201=CARTESIAN_POINT('Ctrl Pts',(0.741647053339758,0.0400023925443897,
6.03352542353788));
#9202=CARTESIAN_POINT('Ctrl Pts',(0.6215856897095,0.429424608756888,6.0606712019436));
#9203=CARTESIAN_POINT('Ctrl Pts',(0.272788863259715,0.708464025234,6.09040985442785));
#9204=CARTESIAN_POINT('Ctrl Pts',(-0.174640201386968,0.742128787355836,
6.12028246378202));
#9205=CARTESIAN_POINT('Ctrl Pts',(-0.565102038705666,0.517026489502915,
6.1502917775661));
#9206=CARTESIAN_POINT('Ctrl Pts',(-0.762043624567604,0.109327312662896,
6.18044350600909));
#9207=CARTESIAN_POINT('Ctrl Pts',(-0.692189456122551,-0.359678326088431,
6.21200701480215));
#9208=CARTESIAN_POINT('Ctrl Pts',(-0.337773460931687,-0.715129603852559,
6.24501197076816));
#9209=CARTESIAN_POINT('Ctrl Pts',(0.124866016940657,-0.767119798247897,
6.27565761479799));
#9210=CARTESIAN_POINT('Ctrl Pts',(0.482663833907203,-0.594530247737682,
6.30260654020584));
#9211=CARTESIAN_POINT('Ctrl Pts',(0.695450511759543,-0.32768100442103,6.32580056862507));
#9212=CARTESIAN_POINT('Ctrl Pts',(0.785412896461935,0.0626075158038052,
6.35297268106789));
#9213=CARTESIAN_POINT('Ctrl Pts',(0.629799785153589,0.510459438093438,6.38419099540486));
#9214=CARTESIAN_POINT('Ctrl Pts',(0.174872432500897,0.796962684150136,6.41953687685404));
#9215=CARTESIAN_POINT('Ctrl Pts',(-0.362484676752387,0.736952725256016,
6.4551134881321));
#9216=CARTESIAN_POINT('Ctrl Pts',(-0.74792746534711,0.35245915978463,6.49092474388711));
#9217=CARTESIAN_POINT('Ctrl Pts',(-0.809887309570728,-0.192065947901566,
6.52697449126839));
#9218=CARTESIAN_POINT('Ctrl Pts',(-0.516915158076634,-0.65954619222211,
6.56326583721123));
#9219=CARTESIAN_POINT('Ctrl Pts',(0.00709632936792426,-0.843579839117015,
6.59980147205316));
#9220=CARTESIAN_POINT('Ctrl Pts',(0.535080054211952,-0.659528972736876,
6.63658345012356));
#9221=CARTESIAN_POINT('Ctrl Pts',(0.834961098454938,-0.183143056575008,
6.67361341976074));
#9222=CARTESIAN_POINT('Ctrl Pts',(0.772836475154942,0.379911298835229,6.71089252375131));
#9223=CARTESIAN_POINT('Ctrl Pts',(0.369319867823668,0.784090370590367,6.74842072124706));
#9224=CARTESIAN_POINT('Ctrl Pts',(-0.137507651352654,0.841177037621035,
6.78200064499767));
#9225=CARTESIAN_POINT('Ctrl Pts',(-0.529655686323561,0.651783755111279,
6.81154496618753));
#9226=CARTESIAN_POINT('Ctrl Pts',(-0.763440172149879,0.359289385813127,
6.83697845361481));
#9227=CARTESIAN_POINT('Ctrl Pts',(-0.847211586055085,-0.0075813723717918,
6.86252259094478));
#9228=CARTESIAN_POINT('Ctrl Pts',(-0.763337400290734,-0.37595112739322,
6.88817526440515));
#9229=CARTESIAN_POINT('Ctrl Pts',(-0.526914388323573,-0.672730225787424,
6.91393691075106));
#9230=CARTESIAN_POINT('Ctrl Pts',(-0.183698562689997,-0.838276618909781,
6.93980597887144));
#9231=CARTESIAN_POINT('Ctrl Pts',(0.198889088741007,-0.838335964394735,
6.96578323697683));
#9232=CARTESIAN_POINT('Ctrl Pts',(0.545106947003364,-0.67180754918665,6.99186582148597));
#9233=CARTESIAN_POINT('Ctrl Pts',(0.785703595073577,-0.370406649743822,
7.01805361583897));
#9234=CARTESIAN_POINT('Ctrl Pts',(0.872119316826772,0.00721196141493378,
7.04434542939925));
#9235=CARTESIAN_POINT('Ctrl Pts',(0.785618184490446,0.386004597261683,7.07073989965295));
#9236=CARTESIAN_POINT('Ctrl Pts',(0.502331801959327,0.742799085163601,7.10165209474801));
#9237=CARTESIAN_POINT('Ctrl Pts',(-0.00621863503242753,0.921910367253639,
7.13714527690347));
#9238=CARTESIAN_POINT('Ctrl Pts',(-0.582851103775203,0.720649175322028,
7.17729562502998));
#9239=CARTESIAN_POINT('Ctrl Pts',(-0.909668842554882,0.201440782148561,
7.21765904401918));
#9240=CARTESIAN_POINT('Ctrl Pts',(-0.841213659251149,-0.41162272843365,
7.25823121418976));
#9241=CARTESIAN_POINT('Ctrl Pts',(-0.403262459624705,-0.850227454077078,
7.29900198947476));
#9242=CARTESIAN_POINT('Ctrl Pts',(0.215483513378321,-0.920627886099326,
7.33997190269741));
#9243=CARTESIAN_POINT('Ctrl Pts',(0.745429336505933,-0.587899220267355,
7.3811170115228));
#9244=CARTESIAN_POINT('Ctrl Pts',(0.883871797949062,-0.193227595737394,
7.40868621059601));
#9245=CARTESIAN_POINT('Ctrl Pts',(0.8838985919702,0.0053707753556189,7.42247342039135));
#9246=CARTESIAN_POINT('Ctrl Pts',(0.750293052325257,-0.00715957249020984,
5.50303372536175));
#9247=CARTESIAN_POINT('Ctrl Pts',(0.750270265731315,0.161735352510056,5.51475884548619));
#9248=CARTESIAN_POINT('Ctrl Pts',(0.632695708259348,0.496355890433882,5.53813632129441));
#9249=CARTESIAN_POINT('Ctrl Pts',(0.18381648383294,0.778081359279531,5.57298649818651));
#9250=CARTESIAN_POINT('Ctrl Pts',(-0.339280552431234,0.718378415257623,
5.6076202896276));
#9251=CARTESIAN_POINT('Ctrl Pts',(-0.709001801655557,0.347985187059841,
5.64204689091912));
#9252=CARTESIAN_POINT('Ctrl Pts',(-0.766698885918436,-0.16919180614749,
5.67627188750895));
#9253=CARTESIAN_POINT('Ctrl Pts',(-0.491102255096102,-0.606944769908898,
5.71030250431352));
#9254=CARTESIAN_POINT('Ctrl Pts',(-0.00508600093609879,-0.776552326514125,
5.74414714312887));
#9255=CARTESIAN_POINT('Ctrl Pts',(0.388081485630343,-0.638236893263609,
5.77157703947433));
#9256=CARTESIAN_POINT('Ctrl Pts',(0.596158844376195,-0.412773207290159,
5.79269814069561));
#9257=CARTESIAN_POINT('Ctrl Pts',(0.721744080724043,-0.15346691557969,5.81253217830301));
#9258=CARTESIAN_POINT('Ctrl Pts',(0.721291797138653,0.217701679185308,5.83724463136508));
#9259=CARTESIAN_POINT('Ctrl Pts',(0.492248297398938,0.553560023202817,5.86431639993153));
#9260=CARTESIAN_POINT('Ctrl Pts',(0.166319730891556,0.709798906698298,5.88884215604732));
#9261=CARTESIAN_POINT('Ctrl Pts',(-0.157783238149665,0.709878237357754,
5.9108529793775));
#9262=CARTESIAN_POINT('Ctrl Pts',(-0.449076273551193,0.569337590676698,
5.9328067996584));
#9263=CARTESIAN_POINT('Ctrl Pts',(-0.650064161571041,0.317172677340155,
5.95470251296732));
#9264=CARTESIAN_POINT('Ctrl Pts',(-0.721621885005776,0.00344024431033504,
5.97654562679051));
#9265=CARTESIAN_POINT('Ctrl Pts',(-0.661964542748072,-0.257286466758943,
5.99470556888389));
#9266=CARTESIAN_POINT('Ctrl Pts',(-0.550269179200512,-0.434720760832016,
6.00921182085571));
#9267=CARTESIAN_POINT('Ctrl Pts',(-0.402276742496014,-0.58292974874922,
6.02370295744568));
#9268=CARTESIAN_POINT('Ctrl Pts',(-0.162278225783224,-0.698511519651894,
6.04178723904388));
#9269=CARTESIAN_POINT('Ctrl Pts',(0.15678598762643,-0.698434753182134,6.06344900909546));
#9270=CARTESIAN_POINT('Ctrl Pts',(0.443832361536606,-0.560174670954122,
6.0850728430943));
#9271=CARTESIAN_POINT('Ctrl Pts',(0.641886657484862,-0.311548705127534,
6.10666325451466));
#9272=CARTESIAN_POINT('Ctrl Pts',(0.720903708581916,0.0325797868375459,
6.13061738623125));
#9273=CARTESIAN_POINT('Ctrl Pts',(0.604189885592221,0.409985700434759,6.15692940855218));
#9274=CARTESIAN_POINT('Ctrl Pts',(0.267732283871283,0.678698793729311,6.1855932204343));
#9275=CARTESIAN_POINT('Ctrl Pts',(-0.161176377088454,0.710602415331958,
6.2142207026778));
#9276=CARTESIAN_POINT('Ctrl Pts',(-0.53324499976805,0.49569736156826,6.2428252689349));
#9277=CARTESIAN_POINT('Ctrl Pts',(-0.71970802918005,0.108916638193807,6.27141553040571));
#9278=CARTESIAN_POINT('Ctrl Pts',(-0.653459538269235,-0.333490314335375,
6.30118792123758));
#9279=CARTESIAN_POINT('Ctrl Pts',(-0.320608653043408,-0.666665722932101,
6.33214798295712));
#9280=CARTESIAN_POINT('Ctrl Pts',(0.11110066391128,-0.714779997862643,6.36073732994674));
#9281=CARTESIAN_POINT('Ctrl Pts',(0.443426222920022,-0.554309028733026,
6.38577168766062));
#9282=CARTESIAN_POINT('Ctrl Pts',(0.640332263629123,-0.307185736963075,
6.4072429033775));
#9283=CARTESIAN_POINT('Ctrl Pts',(0.723203970884255,0.0529817392810816,
6.43231277693535));
#9284=CARTESIAN_POINT('Ctrl Pts',(0.579875213873492,0.464421357446747,6.46099511352603));
#9285=CARTESIAN_POINT('Ctrl Pts',(0.163540281833546,0.726164737539782,6.49332268601409));
#9286=CARTESIAN_POINT('Ctrl Pts',(-0.325806422280217,0.671154653749907,
6.52571901232898));
#9287=CARTESIAN_POINT('Ctrl Pts',(-0.675167952131389,0.322177709778464,
6.55819617950246));
#9288=CARTESIAN_POINT('Ctrl Pts',(-0.730838200739421,-0.169856078141101,
6.59076464701581));
#9289=CARTESIAN_POINT('Ctrl Pts',(-0.466820433339978,-0.590588090246883,
6.62343536526493));
#9290=CARTESIAN_POINT('Ctrl Pts',(0.00350996735505748,-0.755486408003205,
6.65621873257887));
#9291=CARTESIAN_POINT('Ctrl Pts',(0.475826092423244,-0.590582675084604,
6.6891250935537));
#9292=CARTESIAN_POINT('Ctrl Pts',(0.743223728972327,-0.165383236018042,
6.72216417731904));
#9293=CARTESIAN_POINT('Ctrl Pts',(0.687732640812107,0.335833673405217,6.75534872287688));
#9294=CARTESIAN_POINT('Ctrl Pts',(0.329161852114402,0.69473766380513,6.78868194987952));
#9295=CARTESIAN_POINT('Ctrl Pts',(-0.120255207878517,0.745235334942848,
6.81845529502086));
#9296=CARTESIAN_POINT('Ctrl Pts',(-0.467524502978826,0.57746640430216,6.84461903462784));
#9297=CARTESIAN_POINT('Ctrl Pts',(-0.674360922287096,0.318638588168112,
6.86712201294724));
#9298=CARTESIAN_POINT('Ctrl Pts',(-0.748404023106268,-0.00575219575844088,
6.88970750051041));
#9299=CARTESIAN_POINT('Ctrl Pts',(-0.674269101945005,-0.331252076513231,
6.91237414913092));
#9300=CARTESIAN_POINT('Ctrl Pts',(-0.465442485762675,-0.593360030871918,
6.93512642552479));
#9301=CARTESIAN_POINT('Ctrl Pts',(-0.162413298418938,-0.73950734230565,
6.95796516185281));
#9302=CARTESIAN_POINT('Ctrl Pts',(0.175299902719076,-0.739551441572441,
6.98089514210305));
#9303=CARTESIAN_POINT('Ctrl Pts',(0.48087309657339,-0.592568368954699,7.00391530912488));
#9304=CARTESIAN_POINT('Ctrl Pts',(0.693231099227059,-0.326542805878524,
7.02702898588934));
#9305=CARTESIAN_POINT('Ctrl Pts',(0.769520632376555,0.00680181224901938,
7.05023795575404));
#9306=CARTESIAN_POINT('Ctrl Pts',(0.693149586424791,0.341276467608696,7.07354385445611));
#9307=CARTESIAN_POINT('Ctrl Pts',(0.442928349106893,0.656453792431941,7.1008495131406));
#9308=CARTESIAN_POINT('Ctrl Pts',(-0.00655006027916784,0.814828143116751,
7.13222145322597));
#9309=CARTESIAN_POINT('Ctrl Pts',(-0.51677651805262,0.636849892039306,7.16774598353412));
#9310=CARTESIAN_POINT('Ctrl Pts',(-0.806409087124653,0.176948274600164,
7.20350474142154));
#9311=CARTESIAN_POINT('Ctrl Pts',(-0.745817965655065,-0.367012141382838,
7.2395023580954));
#9312=CARTESIAN_POINT('Ctrl Pts',(-0.356682875026977,-0.756951656680894,
7.27574101303561));
#9313=CARTESIAN_POINT('Ctrl Pts',(0.194324484528691,-0.819874060139303,
7.3122257656988));
#9314=CARTESIAN_POINT('Ctrl Pts',(0.667449116817723,-0.523027248491166,
7.34895409901446));
#9315=CARTESIAN_POINT('Ctrl Pts',(0.791458463792618,-0.170101188152833,
7.37361186684348));
#9316=CARTESIAN_POINT('Ctrl Pts',(0.791482481276893,0.00791737913227817,
7.38597037371902));
#9317=CARTESIAN_POINT('Ctrl Pts',(0.849598076317196,-0.00712734349710777,
5.50276247098815));
#9318=CARTESIAN_POINT('Ctrl Pts',(0.849572315215897,0.183814720194332,5.51601816019011));
#9319=CARTESIAN_POINT('Ctrl Pts',(0.716484451910036,0.562864504493882,5.5424997573337));
#9320=CARTESIAN_POINT('Ctrl Pts',(0.20809212706776,0.881898014322701,5.58196713633214));
#9321=CARTESIAN_POINT('Ctrl Pts',(-0.384533142466098,0.814321092392168,
5.6212091202806));
#9322=CARTESIAN_POINT('Ctrl Pts',(-0.803342488001547,0.394693505033448,
5.66020880663821));
#9323=CARTESIAN_POINT('Ctrl Pts',(-0.868627634713463,-0.190973266163329,
5.69896909964657));
#9324=CARTESIAN_POINT('Ctrl Pts',(-0.556653040774226,-0.686349150395686,
5.7374846668518));
#9325=CARTESIAN_POINT('Ctrl Pts',(-0.00707997145394115,-0.878014145711534,
5.77575459287924));
#9326=CARTESIAN_POINT('Ctrl Pts',(0.436900544149483,-0.72169954588876,5.80673549990624));
#9327=CARTESIAN_POINT('Ctrl Pts',(0.671606542222444,-0.467350263792894,
5.83056225412086));
#9328=CARTESIAN_POINT('Ctrl Pts',(0.813155385970533,-0.1750292179711,5.85292188205288));
#9329=CARTESIAN_POINT('Ctrl Pts',(0.812540057938428,0.242883178054026,5.88074814557167));
#9330=CARTESIAN_POINT('Ctrl Pts',(0.554998700939117,0.6202772367454,5.91117655608676));
#9331=CARTESIAN_POINT('Ctrl Pts',(0.189304493774159,0.795493011487289,5.93869516979536));
#9332=CARTESIAN_POINT('Ctrl Pts',(-0.173712239990491,0.795504865118224,
5.96335163063203));
#9333=CARTESIAN_POINT('Ctrl Pts',(-0.499345414071431,0.638313353697133,
5.98789731654311));
#9334=CARTESIAN_POINT('Ctrl Pts',(-0.72356068389146,0.356867037202337,6.01233388291633));
#9335=CARTESIAN_POINT('Ctrl Pts',(-0.803163168357719,0.00747357176146625,
6.03666105392709));
#9336=CARTESIAN_POINT('Ctrl Pts',(-0.736797982336716,-0.28222992698738,
6.05684360012597));
#9337=CARTESIAN_POINT('Ctrl Pts',(-0.612891815719577,-0.479031268493863,
6.07293511022899));
#9338=CARTESIAN_POINT('Ctrl Pts',(-0.448917230819194,-0.643222296978376,
6.08899082487842));
#9339=CARTESIAN_POINT('Ctrl Pts',(-0.18345184155449,-0.770972157981274,
6.10899459772628));
#9340=CARTESIAN_POINT('Ctrl Pts',(0.168509519247147,-0.770779631725406,
6.1328926650123));
#9341=CARTESIAN_POINT('Ctrl Pts',(0.484258307101598,-0.618569501699951,
6.15668614964677));
#9342=CARTESIAN_POINT('Ctrl Pts',(0.7014559478794,-0.345739709198507,6.18037560572192));
#9343=CARTESIAN_POINT('Ctrl Pts',(0.787759201210554,0.0307483449030446,
6.20658402952268));
#9344=CARTESIAN_POINT('Ctrl Pts',(0.660297100374137,0.44205148705441,6.23526827245269));
#9345=CARTESIAN_POINT('Ctrl Pts',(0.29489586174265,0.733477282971818,6.2663838499292));
#9346=CARTESIAN_POINT('Ctrl Pts',(-0.168647261234911,0.767641847640704,
6.2973293246475));
#9347=CARTESIAN_POINT('Ctrl Pts',(-0.568727882191308,0.536181820843462,
6.32810567535681));
#9348=CARTESIAN_POINT('Ctrl Pts',(-0.768048251626985,0.121961889290114,
6.35871685457357));
#9349=CARTESIAN_POINT('Ctrl Pts',(-0.697107833504566,-0.349296397819721,
6.39043824166099));
#9350=CARTESIAN_POINT('Ctrl Pts',(-0.344045555812211,-0.701995892428354,
6.42325363059534));
#9351=CARTESIAN_POINT('Ctrl Pts',(0.110773521189623,-0.752235352072163,
6.45337778122228));
#9352=CARTESIAN_POINT('Ctrl Pts',(0.458965638454581,-0.583886825258837,
6.47961716649731));
#9353=CARTESIAN_POINT('Ctrl Pts',(0.664381883487217,-0.325864755846388,
6.50203114286227));
#9354=CARTESIAN_POINT('Ctrl Pts',(0.750332653299937,0.0485776788759206,
6.52809351690923));
#9355=CARTESIAN_POINT('Ctrl Pts',(0.601674226486008,0.473897649396157,6.55776163974272));
#9356=CARTESIAN_POINT('Ctrl Pts',(0.173613673117217,0.742348086642931,6.59098287751551));
#9357=CARTESIAN_POINT('Ctrl Pts',(-0.3258350440189,0.685649541287933,6.62406030334558));
#9358=CARTESIAN_POINT('Ctrl Pts',(-0.679731238547397,0.331354382468774,
6.65700275666622));
#9359=CARTESIAN_POINT('Ctrl Pts',(-0.735255898447251,-0.164397347346024,
6.6898206739066));
#9360=CARTESIAN_POINT('Ctrl Pts',(-0.470558029977308,-0.585159244984441,
6.7225241569716));
#9361=CARTESIAN_POINT('Ctrl Pts',(-0.00278192751448173,-0.748569972495831,
6.75512382817215));
#9362=CARTESIAN_POINT('Ctrl Pts',(0.46350519113553,-0.58518407843876,6.78763042208935));
#9363=CARTESIAN_POINT('Ctrl Pts',(0.725410474458316,-0.167706567477984,
6.82005514647598));
#9364=CARTESIAN_POINT('Ctrl Pts',(0.670774587918448,0.320804047707368,6.85240545447397));
#9365=CARTESIAN_POINT('Ctrl Pts',(0.323092957157568,0.668041717311718,6.88470045447928));
#9366=CARTESIAN_POINT('Ctrl Pts',(-0.109494451463983,0.716184576245998,
6.91336373465137));
#9367=CARTESIAN_POINT('Ctrl Pts',(-0.44188826662967,0.555407233522295,6.93841735921765));
#9368=CARTESIAN_POINT('Ctrl Pts',(-0.639012403336459,0.308500858246645,
6.95988071793453));
#9369=CARTESIAN_POINT('Ctrl Pts',(-0.709192507424316,0.00040641570270789,
6.98133136104379));
#9370=CARTESIAN_POINT('Ctrl Pts',(-0.638918625948615,-0.307487189319304,
7.00277862675193));
#9371=CARTESIAN_POINT('Ctrl Pts',(-0.442028652642433,-0.554399048208452,
7.02422233485342));
#9372=CARTESIAN_POINT('Ctrl Pts',(-0.157482946544586,-0.691481626684627,
7.0456683320825));
#9373=CARTESIAN_POINT('Ctrl Pts',(0.15835851542768,-0.691398914091788,7.06711532573104));
#9374=CARTESIAN_POINT('Ctrl Pts',(0.44307547960184,-0.554307235545146,7.08857226527194));
#9375=CARTESIAN_POINT('Ctrl Pts',(0.64018584092255,-0.307192493791569,7.11004002498397));
#9376=CARTESIAN_POINT('Ctrl Pts',(0.71067332605218,0.00132671397574847,
7.13152214083118));
#9377=CARTESIAN_POINT('Ctrl Pts',(0.640127181409651,0.309809306958141,7.15302225181439));
#9378=CARTESIAN_POINT('Ctrl Pts',(0.409965562319378,0.59950154513597,7.1781297331652));
#9379=CARTESIAN_POINT('Ctrl Pts',(-0.00180430761257666,0.744250295435473,
7.20686838534354));
#9380=CARTESIAN_POINT('Ctrl Pts',(-0.46689999412445,0.581628177637233,7.23926440850474));
#9381=CARTESIAN_POINT('Ctrl Pts',(-0.729602505011613,0.163869023223047,
7.27173917712393));
#9382=CARTESIAN_POINT('Ctrl Pts',(-0.674485616164893,-0.328104186907804,
7.3043020520652));
#9383=CARTESIAN_POINT('Ctrl Pts',(-0.32358572160231,-0.679299557613987,
7.33696613118188));
#9384=CARTESIAN_POINT('Ctrl Pts',(0.171370920939519,-0.735610678055291,
7.36973771478191));
#9385=CARTESIAN_POINT('Ctrl Pts',(0.594929256360531,-0.469509634858928,
7.40263639340595));
#9386=CARTESIAN_POINT('Ctrl Pts',(0.705563583847616,-0.154509464242322,
7.42464584593578));
#9387=CARTESIAN_POINT('Ctrl Pts',(0.705585033709163,0.00447777927316105,
7.4356831493591));
#9388=CARTESIAN_POINT('Ctrl Pts',(0.911787311372316,-0.00175313599507732,
5.42547035947661));
#9389=CARTESIAN_POINT('Ctrl Pts',(0.911759679946333,0.203051830949188,5.43968844708048));
#9390=CARTESIAN_POINT('Ctrl Pts',(0.768907437119982,0.61071591344494,5.46816718430648));
#9391=CARTESIAN_POINT('Ctrl Pts',(0.220284165601068,0.955502366817236,5.51077805671262));
#9392=CARTESIAN_POINT('Ctrl Pts',(-0.422243656323184,0.882710139668278,
5.55332558349325));
#9393=CARTESIAN_POINT('Ctrl Pts',(-0.878386039542625,0.426289581625414,
5.5957765844892));
#9394=CARTESIAN_POINT('Ctrl Pts',(-0.950141006447777,-0.213553723589873,
5.63813025439539));
#9395=CARTESIAN_POINT('Ctrl Pts',(-0.60835728725253,-0.757014115469509,
5.68037224924266));
#9396=CARTESIAN_POINT('Ctrl Pts',(-0.00366338310403281,-0.968314430281517,
5.72249300107482));
#9397=CARTESIAN_POINT('Ctrl Pts',(0.486718248881734,-0.795970516833383,
5.75670865791863));
#9398=CARTESIAN_POINT('Ctrl Pts',(0.74653021351722,-0.514477549037207,5.78308078863264));
#9399=CARTESIAN_POINT('Ctrl Pts',(0.903446118847398,-0.190511009717507,
5.80786424281498));
#9400=CARTESIAN_POINT('Ctrl Pts',(0.90295145376886,0.273634535370419,5.8387700025228));
#9401=CARTESIAN_POINT('Ctrl Pts',(0.616343546706946,0.693954207986666,5.87265196790731));
#9402=CARTESIAN_POINT('Ctrl Pts',(0.208328450290096,0.889559871552857,5.90335942490417));
#9403=CARTESIAN_POINT('Ctrl Pts',(-0.197431208021256,0.889652469467467,
5.93091996947637));
#9404=CARTESIAN_POINT('Ctrl Pts',(-0.562029250439909,0.713737268348937,
5.95840063131195));
#9405=CARTESIAN_POINT('Ctrl Pts',(-0.813494233574056,0.39820149627948,5.98580131723829));
#9406=CARTESIAN_POINT('Ctrl Pts',(-0.902946074851847,0.0058870464447316,
6.01311843029465));
#9407=CARTESIAN_POINT('Ctrl Pts',(-0.828377509677636,-0.319866751453087,
6.03581174060078));
#9408=CARTESIAN_POINT('Ctrl Pts',(-0.688936970150508,-0.541360820821501,
6.05392170180393));
#9409=CARTESIAN_POINT('Ctrl Pts',(-0.504293132651573,-0.726263454623667,
6.07200206864918));
#9410=CARTESIAN_POINT('Ctrl Pts',(-0.205118119105362,-0.870286210128437,
6.0945471479209));
#9411=CARTESIAN_POINT('Ctrl Pts',(0.191971983732839,-0.870117700265186,
6.12150897978661));
#9412=CARTESIAN_POINT('Ctrl Pts',(0.548553466642107,-0.698273117288175,
6.14837718076188));
#9413=CARTESIAN_POINT('Ctrl Pts',(0.794052616995502,-0.389950825708538,
6.17514969693223));
#9414=CARTESIAN_POINT('Ctrl Pts',(0.891698024550524,0.0358312226908213,
6.20478886300642));
#9415=CARTESIAN_POINT('Ctrl Pts',(0.74749095040922,0.501334011480795,6.23725086378811));
#9416=CARTESIAN_POINT('Ctrl Pts',(0.333743343393983,0.831378563455359,6.27248425191807));
#9417=CARTESIAN_POINT('Ctrl Pts',(-0.19134387466354,0.870105625426578,6.3075348767601));
#9418=CARTESIAN_POINT('Ctrl Pts',(-0.644616547373273,0.607881105022717,
6.34239973374175));
#9419=CARTESIAN_POINT('Ctrl Pts',(-0.870417110421222,0.138612855199806,
6.37707657725051));
#9420=CARTESIAN_POINT('Ctrl Pts',(-0.790048775469081,-0.39510788351932,
6.41299953612703));
#9421=CARTESIAN_POINT('Ctrl Pts',(-0.390383204661376,-0.794274173322802,
6.45013660062964));
#9422=CARTESIAN_POINT('Ctrl Pts',(0.123964069137483,-0.851002982786416,
6.48419818277685));
#9423=CARTESIAN_POINT('Ctrl Pts',(0.517349958215306,-0.660759929294058,
6.51384272570464));
#9424=CARTESIAN_POINT('Ctrl Pts',(0.749191592206741,-0.369479150376496,
6.53914157276564));
#9425=CARTESIAN_POINT('Ctrl Pts',(0.846067098454331,0.052769037404062,6.56852738290555));
#9426=CARTESIAN_POINT('Ctrl Pts',(0.678541487051601,0.531594017531224,6.60192411587722));
#9427=CARTESIAN_POINT('Ctrl Pts',(0.197445708687755,0.833056774682923,6.63924640568331));
#9428=CARTESIAN_POINT('Ctrl Pts',(-0.362407034535075,0.76926077023711,6.67631865996902));
#9429=CARTESIAN_POINT('Ctrl Pts',(-0.757891257853047,0.372960662447378,
6.7131423125874));
#9430=CARTESIAN_POINT('Ctrl Pts',(-0.819502812158925,-0.17971389368945,
6.74971854734871));
#9431=CARTESIAN_POINT('Ctrl Pts',(-0.525117958852971,-0.647082052916212,
6.78604945080241));
#9432=CARTESIAN_POINT('Ctrl Pts',(-0.00706009915885147,-0.827706145589558,
6.82213749402266));
#9433=CARTESIAN_POINT('Ctrl Pts',(0.507168732938518,-0.647142083318005,
6.85798569667506));
#9434=CARTESIAN_POINT('Ctrl Pts',(0.794559460318739,-0.188312585352296,
6.89359746949419));
#9435=CARTESIAN_POINT('Ctrl Pts',(0.734412407851191,0.346047384757273,6.92898046138837));
#9436=CARTESIAN_POINT('Ctrl Pts',(0.35554627917015,0.723799648271606,6.96413145325235));
#9437=CARTESIAN_POINT('Ctrl Pts',(-0.113206435891536,0.775602232806529,
6.99517934888198));
#9438=CARTESIAN_POINT('Ctrl Pts',(-0.471799040782441,0.601968214167806,
7.0222090326148));
#9439=CARTESIAN_POINT('Ctrl Pts',(-0.6836661147338,0.336404243341276,7.04528069450069));
#9440=CARTESIAN_POINT('Ctrl Pts',(-0.758726003996092,0.0062400461075705,
7.06826344122686));
#9441=CARTESIAN_POINT('Ctrl Pts',(-0.6835849590214,-0.322409867084328,7.09115224380289));
#9442=CARTESIAN_POINT('Ctrl Pts',(-0.474072442185209,-0.584919976115439,
7.11395355010067));
#9443=CARTESIAN_POINT('Ctrl Pts',(-0.172560181698569,-0.730020088066619,
7.13666650878931));
#9444=CARTESIAN_POINT('Ctrl Pts',(0.16078217307758,-0.729778328929261,7.15929927954856));
#9445=CARTESIAN_POINT('Ctrl Pts',(0.459989212508115,-0.585545816121325,
7.18184723354721));
#9446=CARTESIAN_POINT('Ctrl Pts',(0.666223161118391,-0.32674631555655,7.20431603435277));
#9447=CARTESIAN_POINT('Ctrl Pts',(0.739554158501798,-0.00504686561265504,
7.22670799379599));
#9448=CARTESIAN_POINT('Ctrl Pts',(0.666159558065311,0.315205418031567,7.24902537021377));
#9449=CARTESIAN_POINT('Ctrl Pts',(0.428020561210259,0.614621005636118,7.27497954766194));
#9450=CARTESIAN_POINT('Ctrl Pts',(0.00440289337514439,0.763018006049135,
7.30452179484735));
#9451=CARTESIAN_POINT('Ctrl Pts',(-0.470624128322024,0.596319364034835,
7.33761244678054));
#9452=CARTESIAN_POINT('Ctrl Pts',(-0.736811683564632,0.171965979607826,
7.37056624676418));
#9453=CARTESIAN_POINT('Ctrl Pts',(-0.68068387352667,-0.324086643305756,
7.4033919913947));
#9454=CARTESIAN_POINT('Ctrl Pts',(-0.328791217341046,-0.675487864461335,
7.43610391008164));
#9455=CARTESIAN_POINT('Ctrl Pts',(0.163774412047771,-0.731012482418632,
7.4687018632077));
#9456=CARTESIAN_POINT('Ctrl Pts',(0.582152961317522,-0.467440680790944,
7.50121977146286));
#9457=CARTESIAN_POINT('Ctrl Pts',(0.690380552641563,-0.158133439986746,
7.52281364669809));
#9458=CARTESIAN_POINT('Ctrl Pts',(0.690401574315868,-0.00231993767140268,
7.53363062084317));
#9459=CARTESIAN_POINT('Ctrl Pts',(0.889359432826132,0.00495444760725769,
5.32880713791624));
#9460=CARTESIAN_POINT('Ctrl Pts',(0.889332447864276,0.204967802847453,5.34269257951066));
#9461=CARTESIAN_POINT('Ctrl Pts',(0.750004347575518,0.603672713614473,5.37053043303203));
#9462=CARTESIAN_POINT('Ctrl Pts',(0.21096706922133,0.94314460394843,5.41241969183905));
#9463=CARTESIAN_POINT('Ctrl Pts',(-0.423963274156834,0.87171349864309,5.45445132266662));
#9464=CARTESIAN_POINT('Ctrl Pts',(-0.877374490363263,0.418799407840054,
5.4966071161887));
#9465=CARTESIAN_POINT('Ctrl Pts',(-0.949545774103564,-0.219892556824646,
5.53888079270843));
#9466=CARTESIAN_POINT('Ctrl Pts',(-0.607068575689537,-0.765494054358749,
5.58125986451715));
#9467=CARTESIAN_POINT('Ctrl Pts',(0.00261167844658479,-0.97913119777945,
5.62373519298684));
#9468=CARTESIAN_POINT('Ctrl Pts',(0.499852533620251,-0.8048463257254,5.65841239967706));
#9469=CARTESIAN_POINT('Ctrl Pts',(0.764265215589788,-0.518466038803169,
5.68524380080038));
#9470=CARTESIAN_POINT('Ctrl Pts',(0.924328881255501,-0.188150671604858,
5.71051448038525));
#9471=CARTESIAN_POINT('Ctrl Pts',(0.924132430512447,0.286757902074732,5.74213409224145));
#9472=CARTESIAN_POINT('Ctrl Pts',(0.62986087869606,0.718937325916808,5.77695468815655));
#9473=CARTESIAN_POINT('Ctrl Pts',(0.208953775300158,0.920912997464213,5.80863418802737));
#9474=CARTESIAN_POINT('Ctrl Pts',(-0.211068988110463,0.921157282542793,
5.83716174516452));
#9475=CARTESIAN_POINT('Ctrl Pts',(-0.589810577699277,0.738585626106938,
5.86570218738055));
#9476=CARTESIAN_POINT('Ctrl Pts',(-0.85194552766839,0.409898301969846,5.89425134138179));
#9477=CARTESIAN_POINT('Ctrl Pts',(-0.945597945878367,-0.000176678256206242,
5.92280607763768));
#9478=CARTESIAN_POINT('Ctrl Pts',(-0.867511729419428,-0.341824865852328,
5.94660339370044));
#9479=CARTESIAN_POINT('Ctrl Pts',(-0.720944780593085,-0.574681060925877,
5.96564071682787));
#9480=CARTESIAN_POINT('Ctrl Pts',(-0.526555141270467,-0.769375552079073,
5.98467700523746));
#9481=CARTESIAN_POINT('Ctrl Pts',(-0.210870756052851,-0.921475670946048,
6.00846936790163));
#9482=CARTESIAN_POINT('Ctrl Pts',(0.209506448294534,-0.921438779399368,
6.03701193615958));
#9483=CARTESIAN_POINT('Ctrl Pts',(0.588220824730041,-0.739083885420811,
6.0655428661009));
#9484=CARTESIAN_POINT('Ctrl Pts',(0.849810718286318,-0.410765395052392,
6.09405857275419));
#9485=CARTESIAN_POINT('Ctrl Pts',(0.95427567990068,0.0440511715684175,6.12572236137368));
#9486=CARTESIAN_POINT('Ctrl Pts',(0.799967960952214,0.54314825140328,6.16052078866217));
#9487=CARTESIAN_POINT('Ctrl Pts',(0.354946991113063,0.898546473402006,6.19843574858538));
#9488=CARTESIAN_POINT('Ctrl Pts',(-0.212199085766547,0.940684954588202,
6.23629684514792));
#9489=CARTESIAN_POINT('Ctrl Pts',(-0.703732454340991,0.656671161576527,
6.27409476897982));
#9490=CARTESIAN_POINT('Ctrl Pts',(-0.949639640621547,0.146281182681,6.31182133692065));
#9491=CARTESIAN_POINT('Ctrl Pts',(-0.862200374710721,-0.436390813484725,
6.35103882924841));
#9492=CARTESIAN_POINT('Ctrl Pts',(-0.424615550503731,-0.87396308504598,
6.39172839424829));
#9493=CARTESIAN_POINT('Ctrl Pts',(0.140875049279472,-0.936660006455991,
6.42918239638723));
#9494=CARTESIAN_POINT('Ctrl Pts',(0.574670287621894,-0.727011014446981,
6.46186903203473));
#9495=CARTESIAN_POINT('Ctrl Pts',(0.83093266790137,-0.405200393190354,6.48982632103455));
#9496=CARTESIAN_POINT('Ctrl Pts',(0.938317766588939,0.0623494789078903,
6.52236975513327));
#9497=CARTESIAN_POINT('Ctrl Pts',(0.752579540678534,0.594055251251905,6.55945509994811));
#9498=CARTESIAN_POINT('Ctrl Pts',(0.217059284541729,0.929973502219806,6.60101727981861));
#9499=CARTESIAN_POINT('Ctrl Pts',(-0.408026785252189,0.859019100893442,
6.6424136299843));
#9500=CARTESIAN_POINT('Ctrl Pts',(-0.850845977716372,0.415638179906151,
6.68363494790014));
#9501=CARTESIAN_POINT('Ctrl Pts',(-0.920184777472661,-0.204329024249146,
6.72467349392044));
#9502=CARTESIAN_POINT('Ctrl Pts',(-0.589428074185655,-0.729814282912527,
6.76552142650441));
#9503=CARTESIAN_POINT('Ctrl Pts',(-0.00604978450581677,-0.933394312826398,
6.80617154371966));
#9504=CARTESIAN_POINT('Ctrl Pts',(0.57404869025302,-0.72985742835735,6.84661700406497));
#9505=CARTESIAN_POINT('Ctrl Pts',(0.898783211561984,-0.211649435517353,
6.8868516259356));
#9506=CARTESIAN_POINT('Ctrl Pts',(0.830853561486015,0.392570978289185,6.92686564614092));
#9507=CARTESIAN_POINT('Ctrl Pts',(0.402102843122056,0.820171632165624,6.96666187541315));
#9508=CARTESIAN_POINT('Ctrl Pts',(-0.128752136760593,0.87885181573823,7.0018337119622));
#9509=CARTESIAN_POINT('Ctrl Pts',(-0.534933891924655,0.682185839564183,
7.03245541763881));
#9510=CARTESIAN_POINT('Ctrl Pts',(-0.774943785493673,0.381327511531892,
7.05860032562784));
#9511=CARTESIAN_POINT('Ctrl Pts',(-0.859966110515312,0.00734177845082202,
7.08463607645075));
#9512=CARTESIAN_POINT('Ctrl Pts',(-0.774831422913684,-0.364904312674865,
7.11056853328824));
#9513=CARTESIAN_POINT('Ctrl Pts',(-0.537583138232402,-0.662143756003773,
7.13639250543407));
#9514=CARTESIAN_POINT('Ctrl Pts',(-0.196279169025999,-0.826362279426242,
7.16211006197668));
#9515=CARTESIAN_POINT('Ctrl Pts',(0.180788904256726,-0.82607059745876,7.18771480491698));
#9516=CARTESIAN_POINT('Ctrl Pts',(0.519038634180724,-0.662978803853832,
7.21321277550856));
#9517=CARTESIAN_POINT('Ctrl Pts',(0.751978439186691,-0.370613914749894,
7.23860036966167));
#9518=CARTESIAN_POINT('Ctrl Pts',(0.834701683971329,-0.00754650688657486,
7.26387733624003));
#9519=CARTESIAN_POINT('Ctrl Pts',(0.751920252216622,0.353483451503403,7.28904368273798));
#9520=CARTESIAN_POINT('Ctrl Pts',(0.483730036422595,0.690590593695916,7.31827398545647));
#9521=CARTESIAN_POINT('Ctrl Pts',(0.00742785048027893,0.857265989116031,
7.35149921639049));
#9522=CARTESIAN_POINT('Ctrl Pts',(-0.525293231887737,0.670073438058683,
7.38862588821794));
#9523=CARTESIAN_POINT('Ctrl Pts',(-0.822869944746703,0.195197072733832,
7.42550481928346));
#9524=CARTESIAN_POINT('Ctrl Pts',(-0.759959606004209,-0.358130855720698,
7.46213543363099));
#9525=CARTESIAN_POINT('Ctrl Pts',(-0.368415214766548,-0.748693330694505,
7.49852208898732));
#9526=CARTESIAN_POINT('Ctrl Pts',(0.177541916017237,-0.809855769006471,
7.53466251134493));
#9527=CARTESIAN_POINT('Ctrl Pts',(0.639295990646259,-0.518615892317653,
7.57056942797824));
#9528=CARTESIAN_POINT('Ctrl Pts',(0.758201052838224,-0.178255309934477,
7.59433715581631));
#9529=CARTESIAN_POINT('Ctrl Pts',(0.758224108327783,-0.00736708650145173,
7.60620065587956));
#9530=CARTESIAN_POINT('Ctrl Pts',(0.829918995390605,0.00692962491070555,
5.30024010712383));
#9531=CARTESIAN_POINT('Ctrl Pts',(0.829893790259993,0.193750817013165,5.31320971482039));
#9532=CARTESIAN_POINT('Ctrl Pts',(0.699822285583035,0.566145381882556,5.3392101566049));
#9533=CARTESIAN_POINT('Ctrl Pts',(0.195323515234371,0.88416117171195,5.37842883489126));
#9534=CARTESIAN_POINT('Ctrl Pts',(-0.400343151138505,0.817346474568011,
5.41785865980122));
#9535=CARTESIAN_POINT('Ctrl Pts',(-0.826817727686594,0.391700174990477,
5.4574958434249));
#9536=CARTESIAN_POINT('Ctrl Pts',(-0.895091678603364,-0.210180305596499,
5.49733544534094));
#9537=CARTESIAN_POINT('Ctrl Pts',(-0.571783532988076,-0.72574941013594,
5.53737192540201));
#9538=CARTESIAN_POINT('Ctrl Pts',(0.00554627097635579,-0.928352383739425,
5.57760056939562));
#9539=CARTESIAN_POINT('Ctrl Pts',(0.477799679854192,-0.76307476144334,5.61052921806703));
#9540=CARTESIAN_POINT('Ctrl Pts',(0.729410852594162,-0.490616169914011,
5.63605789108779));
#9541=CARTESIAN_POINT('Ctrl Pts',(0.881919476817548,-0.175979128010471,
5.66013043243701));
#9542=CARTESIAN_POINT('Ctrl Pts',(0.881906152444497,0.277265930526209,5.69030700929344));
#9543=CARTESIAN_POINT('Ctrl Pts',(0.600514890488868,0.690886371812261,5.72362170442843));
#9544=CARTESIAN_POINT('Ctrl Pts',(0.196921477412404,0.884675277260858,5.75399952860311));
#9545=CARTESIAN_POINT('Ctrl Pts',(-0.206656190820974,0.885009407611865,
5.78140796402136));
#9546=CARTESIAN_POINT('Ctrl Pts',(-0.571352525906284,0.709312471916405,
5.80888598178339));
#9547=CARTESIAN_POINT('Ctrl Pts',(-0.824322784093117,0.39228222278969,5.8364255516956));
#9548=CARTESIAN_POINT('Ctrl Pts',(-0.914955919505048,-0.00412326864883124,
5.86402777825679));
#9549=CARTESIAN_POINT('Ctrl Pts',(-0.839394814319228,-0.335102288993869,
5.88707765903504));
#9550=CARTESIAN_POINT('Ctrl Pts',(-0.697194784237861,-0.561053925833896,
5.90554855730548));
#9551=CARTESIAN_POINT('Ctrl Pts',(-0.508394551716055,-0.75017609097147,
5.9240379575655));
#9552=CARTESIAN_POINT('Ctrl Pts',(-0.201331843767861,-0.89822223947356,
5.94717992736717));
#9553=CARTESIAN_POINT('Ctrl Pts',(0.208503775368862,-0.898293333883727,
5.97500361673599));
#9554=CARTESIAN_POINT('Ctrl Pts',(0.578566181754719,-0.72022509709185,6.00287494476189));
#9555=CARTESIAN_POINT('Ctrl Pts',(0.834785028018541,-0.398807815817064,
6.03079323532));
#9556=CARTESIAN_POINT('Ctrl Pts',(0.937421618538533,0.0474693145637866,
6.06185942553353));
#9557=CARTESIAN_POINT('Ctrl Pts',(0.785808706512713,0.53858289651246,6.09609235737173));
#9558=CARTESIAN_POINT('Ctrl Pts',(0.346833476768302,0.889498241929319,6.13350258691761));
#9559=CARTESIAN_POINT('Ctrl Pts',(-0.214450953963022,0.931459250732699,
6.17096335002368));
#9560=CARTESIAN_POINT('Ctrl Pts',(-0.702523232936964,0.649744126672763,
6.20847735887153));
#9561=CARTESIAN_POINT('Ctrl Pts',(-0.947620032703892,0.141637172177686,
6.24603852533507));
#9562=CARTESIAN_POINT('Ctrl Pts',(-0.860569087705711,-0.440346323520561,
6.28520072180747));
#9563=CARTESIAN_POINT('Ctrl Pts',(-0.422417509108382,-0.879011958721694,
6.32595508450303));
#9564=CARTESIAN_POINT('Ctrl Pts',(0.146053510149855,-0.942361769529175,
6.36359784749923));
#9565=CARTESIAN_POINT('Ctrl Pts',(0.583529811691089,-0.731092224974979,
6.39655251871174));
#9566=CARTESIAN_POINT('Ctrl Pts',(0.842579028174264,-0.405926837413371,
6.42480144817265));
#9567=CARTESIAN_POINT('Ctrl Pts',(0.951487177832284,0.0675991994034292,
6.45775864234018));
#9568=CARTESIAN_POINT('Ctrl Pts',(0.763141746082221,0.607725575505774,6.49541116932488));
#9569=CARTESIAN_POINT('Ctrl Pts',(0.217574487524898,0.950392778021499,6.53775763542001));
#9570=CARTESIAN_POINT('Ctrl Pts',(-0.42166740973873,0.878191572890031,6.58007504544765));
#9571=CARTESIAN_POINT('Ctrl Pts',(-0.876250398231941,0.423545215383675,
6.62235503675604));
#9572=CARTESIAN_POINT('Ctrl Pts',(-0.947987096499237,-0.21459643925478,
6.6645859298645));
#9573=CARTESIAN_POINT('Ctrl Pts',(-0.606705076713124,-0.757473932422971,
6.70675774894366));
#9574=CARTESIAN_POINT('Ctrl Pts',(-0.00241202776964925,-0.968727997454768,
6.74885991888449));
#9575=CARTESIAN_POINT('Ctrl Pts',(0.600624482148029,-0.757509613558942,
6.79088237303874));
#9576=CARTESIAN_POINT('Ctrl Pts',(0.939452177122731,-0.217421016410473,
6.8328144749144));
#9577=CARTESIAN_POINT('Ctrl Pts',(0.868758799747721,0.414536277515111,6.87465507197778));
#9578=CARTESIAN_POINT('Ctrl Pts',(0.419290549746345,0.863247184920627,6.91637647714826));
#9579=CARTESIAN_POINT('Ctrl Pts',(-0.139084650191804,0.925265402913614,
6.95335818017224));
#9580=CARTESIAN_POINT('Ctrl Pts',(-0.567454545740675,0.717965354424563,
6.98564100520883));
#9581=CARTESIAN_POINT('Ctrl Pts',(-0.821064769263926,0.400211556185252,
7.0132490098583));
#9582=CARTESIAN_POINT('Ctrl Pts',(-0.91112933929112,0.00438963293201363,
7.04080231652177));
#9583=CARTESIAN_POINT('Ctrl Pts',(-0.820966778853315,-0.390275853878312,
7.0682856755789));
#9584=CARTESIAN_POINT('Ctrl Pts',(-0.569057996064222,-0.706001271167066,
7.09570447796615));
#9585=CARTESIAN_POINT('Ctrl Pts',(-0.206027274734066,-0.880764451318613,
7.1230513221731));
#9586=CARTESIAN_POINT('Ctrl Pts',(0.195812674813625,-0.880515195886687,
7.15033395522949));
#9587=CARTESIAN_POINT('Ctrl Pts',(0.556847139748695,-0.706517914293179,
7.17753857633508));
#9588=CARTESIAN_POINT('Ctrl Pts',(0.805895709935206,-0.394032847218828,
7.20466842663578));
#9589=CARTESIAN_POINT('Ctrl Pts',(0.894511398596212,-0.00535918267020315,
7.2317212151674));
#9590=CARTESIAN_POINT('Ctrl Pts',(0.805810304168001,0.381721934163946,7.25869451527825));
#9591=CARTESIAN_POINT('Ctrl Pts',(0.517921324180488,0.743697104768732,7.29007024661223));
#9592=CARTESIAN_POINT('Ctrl Pts',(0.00578604455006559,0.923078227892816,
7.32578329054371));
#9593=CARTESIAN_POINT('Ctrl Pts',(-0.568243145767641,0.721567999099011,
7.3657709938243));
#9594=CARTESIAN_POINT('Ctrl Pts',(-0.889554950114489,0.209118291781916,
7.40555959496073));
#9595=CARTESIAN_POINT('Ctrl Pts',(-0.821710123582801,-0.38904286980981,
7.44514503289073));
#9596=CARTESIAN_POINT('Ctrl Pts',(-0.397947019918738,-0.811956407468429,
7.48452302388204));
#9597=CARTESIAN_POINT('Ctrl Pts',(0.193792979174468,-0.878334837234862,
7.52368670026048));
#9598=CARTESIAN_POINT('Ctrl Pts',(0.694889984053186,-0.562420176620936,
7.56263844726097));
#9599=CARTESIAN_POINT('Ctrl Pts',(0.823996878593897,-0.192605752293447,
7.58845159102269));
#9600=CARTESIAN_POINT('Ctrl Pts',(0.824021914564924,-0.00703811992170032,
7.60133417341575));
#9601=CARTESIAN_POINT('Ctrl Pts',(0.799999065628721,0.00692558823944229,
5.30024010712383));
#9602=CARTESIAN_POINT('Ctrl Pts',(0.799974755250737,0.187114846749742,5.31274930893178));
#9603=CARTESIAN_POINT('Ctrl Pts',(0.674578200671659,0.546127076651831,5.33781512365923));
#9604=CARTESIAN_POINT('Ctrl Pts',(0.187998995393781,0.852903359039399,5.37564381521248));
#9605=CARTESIAN_POINT('Ctrl Pts',(-0.386721866921525,0.788448388841122,
5.41368605209984));
#9606=CARTESIAN_POINT('Ctrl Pts',(-0.7983994419892,0.377627224111744,5.45194644400096));
#9607=CARTESIAN_POINT('Ctrl Pts',(-0.864375113399524,-0.203617876612744,
5.49042055747836));
#9608=CARTESIAN_POINT('Ctrl Pts',(-0.552019639313923,-0.701812288635587,
5.52910737914477));
#9609=CARTESIAN_POINT('Ctrl Pts',(0.00615426428515267,-0.897757418326962,
5.56800374230524));
#9610=CARTESIAN_POINT('Ctrl Pts',(0.463089276607972,-0.737891299975203,
5.59986549204054));
#9611=CARTESIAN_POINT('Ctrl Pts',(0.706662565433678,-0.474149107376678,
5.62457829573124));
#9612=CARTESIAN_POINT('Ctrl Pts',(0.854347338563578,-0.169471123140589,
5.6478904398873));
#9613=CARTESIAN_POINT('Ctrl Pts',(0.854381411403854,0.269671075667267,5.67712918390586));
#9614=CARTESIAN_POINT('Ctrl Pts',(0.581578462406747,0.670744438556907,5.70943359497258));
#9615=CARTESIAN_POINT('Ctrl Pts',(0.189982000930166,0.858805851522918,5.73891161848027));
#9616=CARTESIAN_POINT('Ctrl Pts',(-0.201854620920769,0.859148371452269,
5.76552549972421));
#9617=CARTESIAN_POINT('Ctrl Pts',(-0.556170302204947,0.688486751453872,
5.79222147180784));
#9618=CARTESIAN_POINT('Ctrl Pts',(-0.802120584542054,0.380288702719923,
5.81899788702529));
#9619=CARTESIAN_POINT('Ctrl Pts',(-0.890321102734134,-0.0053444036833259,
5.84585301727138));
#9620=CARTESIAN_POINT('Ctrl Pts',(-0.816781798992104,-0.327577127496462,
5.86829638740099));
#9621=CARTESIAN_POINT('Ctrl Pts',(-0.678277859648778,-0.547664335405585,
5.88628859994389));
#9622=CARTESIAN_POINT('Ctrl Pts',(-0.494316135451619,-0.731945478665225,
5.90430550175064));
#9623=CARTESIAN_POINT('Ctrl Pts',(-0.194941007989142,-0.876310026230692,
5.92687230420244));
#9624=CARTESIAN_POINT('Ctrl Pts',(0.204945568353256,-0.876409485122255,
5.95402353339188));
#9625=CARTESIAN_POINT('Ctrl Pts',(0.566325487118899,-0.702556101088839,
5.98124373289334));
#9626=CARTESIAN_POINT('Ctrl Pts',(0.816751045229916,-0.388463305588866,
6.00853075028047));
#9627=CARTESIAN_POINT('Ctrl Pts',(0.917174982875959,0.0480250206861584,
6.03892142694837));
#9628=CARTESIAN_POINT('Ctrl Pts',(0.768829350780382,0.528866010776267,6.07244001895545));
#9629=CARTESIAN_POINT('Ctrl Pts',(0.338627495917749,0.872873034891815,6.10911095186911));
#9630=CARTESIAN_POINT('Ctrl Pts',(-0.212178222814091,0.914151313349766,
6.14588130840082));
#9631=CARTESIAN_POINT('Ctrl Pts',(-0.691759933067223,0.637451614256161,
6.18274515756461));
#9632=CARTESIAN_POINT('Ctrl Pts',(-0.932934482256533,0.137697594997002,
6.21969639210087));
#9633=CARTESIAN_POINT('Ctrl Pts',(-0.84730393945114,-0.435496308403701,
6.25827178793966));
#9634=CARTESIAN_POINT('Ctrl Pts',(-0.415273257958933,-0.868240176171726,
6.29847623644814));
#9635=CARTESIAN_POINT('Ctrl Pts',(0.146189896678077,-0.930950222024402,
6.33566388079779));
#9636=CARTESIAN_POINT('Ctrl Pts',(0.578787425776111,-0.722091726547751,
6.36825221458814));
#9637=CARTESIAN_POINT('Ctrl Pts',(0.835229259505866,-0.400278931762148,
6.3962159259868));
#9638=CARTESIAN_POINT('Ctrl Pts',(0.943177486850013,0.0688606453452641,
6.42887288667825));
#9639=CARTESIAN_POINT('Ctrl Pts',(0.756462512495389,0.604750444420971,6.46623690685835));
#9640=CARTESIAN_POINT('Ctrl Pts',(0.214509054547464,0.945343920852135,6.50831791566041));
#9641=CARTESIAN_POINT('Ctrl Pts',(-0.421585054233784,0.873670673138226,
6.55043539297339));
#9642=CARTESIAN_POINT('Ctrl Pts',(-0.874725713994987,0.420703846750279,
6.59257924943873));
#9643=CARTESIAN_POINT('Ctrl Pts',(-0.946491736933492,-0.216206220818672,
6.63473932973225));
#9644=CARTESIAN_POINT('Ctrl Pts',(-0.605472064685913,-0.758979181442101,
6.67690544450194));
#9645=CARTESIAN_POINT('Ctrl Pts',(-0.000509641250504898,-0.970641038681315,
6.71906739492544));
#9646=CARTESIAN_POINT('Ctrl Pts',(0.604236817182525,-0.758999928674301,
6.76121498571335));
#9647=CARTESIAN_POINT('Ctrl Pts',(0.944676427167983,-0.216670516455945,
6.80333805746961));
#9648=CARTESIAN_POINT('Ctrl Pts',(0.873719648783539,0.418956634979468,6.8454265042638));
#9649=CARTESIAN_POINT('Ctrl Pts',(0.421037273012308,0.871132652579719,6.88747029453994));
#9650=CARTESIAN_POINT('Ctrl Pts',(-0.142342851291253,0.933831870869633,
6.92479402146672));
#9651=CARTESIAN_POINT('Ctrl Pts',(-0.575104466317865,0.724476767443434,
6.95741054274359));
#9652=CARTESIAN_POINT('Ctrl Pts',(-0.831597121038275,0.403171008458228,
6.98533606563364));
#9653=CARTESIAN_POINT('Ctrl Pts',(-0.922808904665035,0.00254068286457492,
7.01322724854536));
#9654=CARTESIAN_POINT('Ctrl Pts',(-0.831484359832733,-0.397369041930912,
7.04108128388358));
#9655=CARTESIAN_POINT('Ctrl Pts',(-0.576024516479058,-0.717622866946566,
7.06889539860548));
#9656=CARTESIAN_POINT('Ctrl Pts',(-0.207464718971416,-0.895095126308869,
7.09666685370961));
#9657=CARTESIAN_POINT('Ctrl Pts',(0.200869050822812,-0.894893573965507,
7.12439296344474));
#9658=CARTESIAN_POINT('Ctrl Pts',(0.568135301656786,-0.717941543510051,
7.15207107099507));
#9659=CARTESIAN_POINT('Ctrl Pts',(0.821742493579341,-0.399813712939291,
7.17969857736332));
#9660=CARTESIAN_POINT('Ctrl Pts',(0.912100647381109,-0.00372699171446918,
7.20727292857109));
#9661=CARTESIAN_POINT('Ctrl Pts',(0.821667160899362,0.391120281113409,7.23479162069698));
#9662=CARTESIAN_POINT('Ctrl Pts',(0.527798142032111,0.760706416566583,7.26682897888736));
#9663=CARTESIAN_POINT('Ctrl Pts',(0.00437094025093319,0.944184514671381,
7.30334225024583));
#9664=CARTESIAN_POINT('Ctrl Pts',(-0.583164611559206,0.738086874931468,
7.3442757526392));
#9665=CARTESIAN_POINT('Ctrl Pts',(-0.912546668924433,0.213026529714121,
7.38505770065783));
#9666=CARTESIAN_POINT('Ctrl Pts',(-0.843060529623956,-0.400706652853849,
7.42568118182012));
#9667=CARTESIAN_POINT('Ctrl Pts',(-0.407835437985135,-0.835237258109269,
7.46613873367218));
#9668=CARTESIAN_POINT('Ctrl Pts',(0.200737244244076,-0.903598468057941,
7.5064251969444));
#9669=CARTESIAN_POINT('Ctrl Pts',(0.71672352100227,-0.578479045751934,7.54653146106904));
#9670=CARTESIAN_POINT('Ctrl Pts',(0.849917343436364,-0.197265324952655,
7.57314919120958));
#9671=CARTESIAN_POINT('Ctrl Pts',(0.849943147209423,-0.00600671278230411,
7.58642685605973));
#9672=CARTESIAN_POINT('',(0.799999065628721,0.00692558823944227,5.30024010712383));
#9673=CARTESIAN_POINT('Origin',(0.8,-5.53479071733669E-17,5.4));
#9674=CARTESIAN_POINT('',(0.849943147209423,-0.00600671278230414,7.58642685605973));
#9675=CARTESIAN_POINT('Ctrl Pts',(0.799999065628721,0.00692558823944229,
5.30024010712383));
#9676=CARTESIAN_POINT('Ctrl Pts',(0.799974755250737,0.187114846749742,5.31274930893178));
#9677=CARTESIAN_POINT('Ctrl Pts',(0.674578200671659,0.546127076651831,5.33781512365923));
#9678=CARTESIAN_POINT('Ctrl Pts',(0.187998995393781,0.852903359039399,5.37564381521248));
#9679=CARTESIAN_POINT('Ctrl Pts',(-0.386721866921525,0.788448388841122,
5.41368605209984));
#9680=CARTESIAN_POINT('Ctrl Pts',(-0.7983994419892,0.377627224111744,5.45194644400096));
#9681=CARTESIAN_POINT('Ctrl Pts',(-0.864375113399524,-0.203617876612744,
5.49042055747836));
#9682=CARTESIAN_POINT('Ctrl Pts',(-0.552019639313923,-0.701812288635587,
5.52910737914477));
#9683=CARTESIAN_POINT('Ctrl Pts',(0.00615426428515267,-0.897757418326962,
5.56800374230524));
#9684=CARTESIAN_POINT('Ctrl Pts',(0.463089276607972,-0.737891299975203,
5.59986549204054));
#9685=CARTESIAN_POINT('Ctrl Pts',(0.706662565433678,-0.474149107376678,
5.62457829573124));
#9686=CARTESIAN_POINT('Ctrl Pts',(0.854347338563578,-0.169471123140589,
5.6478904398873));
#9687=CARTESIAN_POINT('Ctrl Pts',(0.854381411403854,0.269671075667267,5.67712918390586));
#9688=CARTESIAN_POINT('Ctrl Pts',(0.581578462406747,0.670744438556907,5.70943359497258));
#9689=CARTESIAN_POINT('Ctrl Pts',(0.189982000930166,0.858805851522918,5.73891161848027));
#9690=CARTESIAN_POINT('Ctrl Pts',(-0.201854620920769,0.859148371452269,
5.76552549972421));
#9691=CARTESIAN_POINT('Ctrl Pts',(-0.556170302204947,0.688486751453872,
5.79222147180784));
#9692=CARTESIAN_POINT('Ctrl Pts',(-0.802120584542054,0.380288702719923,
5.81899788702529));
#9693=CARTESIAN_POINT('Ctrl Pts',(-0.890321102734134,-0.0053444036833259,
5.84585301727138));
#9694=CARTESIAN_POINT('Ctrl Pts',(-0.816781798992104,-0.327577127496462,
5.86829638740099));
#9695=CARTESIAN_POINT('Ctrl Pts',(-0.678277859648778,-0.547664335405585,
5.88628859994389));
#9696=CARTESIAN_POINT('Ctrl Pts',(-0.494316135451619,-0.731945478665225,
5.90430550175064));
#9697=CARTESIAN_POINT('Ctrl Pts',(-0.194941007989142,-0.876310026230692,
5.92687230420244));
#9698=CARTESIAN_POINT('Ctrl Pts',(0.204945568353256,-0.876409485122255,
5.95402353339188));
#9699=CARTESIAN_POINT('Ctrl Pts',(0.566325487118899,-0.702556101088839,
5.98124373289334));
#9700=CARTESIAN_POINT('Ctrl Pts',(0.816751045229916,-0.388463305588866,
6.00853075028047));
#9701=CARTESIAN_POINT('Ctrl Pts',(0.917174982875959,0.0480250206861584,
6.03892142694837));
#9702=CARTESIAN_POINT('Ctrl Pts',(0.768829350780382,0.528866010776267,6.07244001895545));
#9703=CARTESIAN_POINT('Ctrl Pts',(0.338627495917749,0.872873034891815,6.10911095186911));
#9704=CARTESIAN_POINT('Ctrl Pts',(-0.212178222814091,0.914151313349766,
6.14588130840082));
#9705=CARTESIAN_POINT('Ctrl Pts',(-0.691759933067223,0.637451614256161,
6.18274515756461));
#9706=CARTESIAN_POINT('Ctrl Pts',(-0.932934482256533,0.137697594997002,
6.21969639210087));
#9707=CARTESIAN_POINT('Ctrl Pts',(-0.84730393945114,-0.435496308403701,
6.25827178793966));
#9708=CARTESIAN_POINT('Ctrl Pts',(-0.415273257958933,-0.868240176171726,
6.29847623644814));
#9709=CARTESIAN_POINT('Ctrl Pts',(0.146189896678077,-0.930950222024402,
6.33566388079779));
#9710=CARTESIAN_POINT('Ctrl Pts',(0.578787425776111,-0.722091726547751,
6.36825221458814));
#9711=CARTESIAN_POINT('Ctrl Pts',(0.835229259505866,-0.400278931762148,
6.3962159259868));
#9712=CARTESIAN_POINT('Ctrl Pts',(0.943177486850013,0.0688606453452641,
6.42887288667825));
#9713=CARTESIAN_POINT('Ctrl Pts',(0.756462512495389,0.604750444420971,6.46623690685835));
#9714=CARTESIAN_POINT('Ctrl Pts',(0.214509054547464,0.945343920852135,6.50831791566041));
#9715=CARTESIAN_POINT('Ctrl Pts',(-0.421585054233784,0.873670673138226,
6.55043539297339));
#9716=CARTESIAN_POINT('Ctrl Pts',(-0.874725713994987,0.420703846750279,
6.59257924943873));
#9717=CARTESIAN_POINT('Ctrl Pts',(-0.946491736933492,-0.216206220818672,
6.63473932973225));
#9718=CARTESIAN_POINT('Ctrl Pts',(-0.605472064685913,-0.758979181442101,
6.67690544450194));
#9719=CARTESIAN_POINT('Ctrl Pts',(-0.000509641250504898,-0.970641038681315,
6.71906739492544));
#9720=CARTESIAN_POINT('Ctrl Pts',(0.604236817182525,-0.758999928674301,
6.76121498571335));
#9721=CARTESIAN_POINT('Ctrl Pts',(0.944676427167983,-0.216670516455945,
6.80333805746961));
#9722=CARTESIAN_POINT('Ctrl Pts',(0.873719648783539,0.418956634979468,6.8454265042638));
#9723=CARTESIAN_POINT('Ctrl Pts',(0.421037273012308,0.871132652579719,6.88747029453994));
#9724=CARTESIAN_POINT('Ctrl Pts',(-0.142342851291253,0.933831870869633,
6.92479402146672));
#9725=CARTESIAN_POINT('Ctrl Pts',(-0.575104466317865,0.724476767443434,
6.95741054274359));
#9726=CARTESIAN_POINT('Ctrl Pts',(-0.831597121038275,0.403171008458228,
6.98533606563364));
#9727=CARTESIAN_POINT('Ctrl Pts',(-0.922808904665035,0.00254068286457492,
7.01322724854536));
#9728=CARTESIAN_POINT('Ctrl Pts',(-0.831484359832733,-0.397369041930912,
7.04108128388358));
#9729=CARTESIAN_POINT('Ctrl Pts',(-0.576024516479058,-0.717622866946566,
7.06889539860548));
#9730=CARTESIAN_POINT('Ctrl Pts',(-0.207464718971416,-0.895095126308869,
7.09666685370961));
#9731=CARTESIAN_POINT('Ctrl Pts',(0.200869050822812,-0.894893573965507,
7.12439296344474));
#9732=CARTESIAN_POINT('Ctrl Pts',(0.568135301656786,-0.717941543510051,
7.15207107099507));
#9733=CARTESIAN_POINT('Ctrl Pts',(0.821742493579341,-0.399813712939291,
7.17969857736332));
#9734=CARTESIAN_POINT('Ctrl Pts',(0.912100647381109,-0.00372699171446918,
7.20727292857109));
#9735=CARTESIAN_POINT('Ctrl Pts',(0.821667160899362,0.391120281113409,7.23479162069698));
#9736=CARTESIAN_POINT('Ctrl Pts',(0.527798142032111,0.760706416566583,7.26682897888736));
#9737=CARTESIAN_POINT('Ctrl Pts',(0.00437094025093319,0.944184514671381,
7.30334225024583));
#9738=CARTESIAN_POINT('Ctrl Pts',(-0.583164611559206,0.738086874931468,
7.3442757526392));
#9739=CARTESIAN_POINT('Ctrl Pts',(-0.912546668924433,0.213026529714121,
7.38505770065783));
#9740=CARTESIAN_POINT('Ctrl Pts',(-0.843060529623956,-0.400706652853849,
7.42568118182012));
#9741=CARTESIAN_POINT('Ctrl Pts',(-0.407835437985135,-0.835237258109269,
7.46613873367218));
#9742=CARTESIAN_POINT('Ctrl Pts',(0.200737244244076,-0.903598468057941,
7.5064251969444));
#9743=CARTESIAN_POINT('Ctrl Pts',(0.71672352100227,-0.578479045751934,7.54653146106904));
#9744=CARTESIAN_POINT('Ctrl Pts',(0.849917343436364,-0.197265324952655,
7.57314919120958));
#9745=CARTESIAN_POINT('Ctrl Pts',(0.849943147209423,-0.00600671278230411,
7.58642685605973));
#9746=CARTESIAN_POINT('Origin',(0.799999999999999,-1.22124532708767E-15,
7.5));
#9747=CARTESIAN_POINT('Origin',(0.799999999999999,-1.22124532708767E-15,
7.5));
#9748=CARTESIAN_POINT('Origin',(0.8,-5.53479071733669E-17,5.4));
#10230=UNCERTAINTY_MEASURE_WITH_UNIT(LENGTH_MEASURE(0.001),#10267,
'DISTANCE_ACCURACY_VALUE',
'Maximum model space distance between geometric entities at asserted c
onnectivities');
#10241=UNCERTAINTY_MEASURE_WITH_UNIT(LENGTH_MEASURE(0.001),#10267,
'DISTANCE_ACCURACY_VALUE',
'Maximum model space distance between geometric entities at asserted c
onnectivities');
#10255=(
GEOMETRIC_REPRESENTATION_CONTEXT(3)
GLOBAL_UNCERTAINTY_ASSIGNED_CONTEXT((#10230))
GLOBAL_UNIT_ASSIGNED_CONTEXT((#10267,#10269,#10270))
REPRESENTATION_CONTEXT('','3D')
);
#10266=(
GEOMETRIC_REPRESENTATION_CONTEXT(3)
GLOBAL_UNCERTAINTY_ASSIGNED_CONTEXT((#10241))
GLOBAL_UNIT_ASSIGNED_CONTEXT((#10267,#10269,#10270))
REPRESENTATION_CONTEXT('','3D')
);
#10267=(
LENGTH_UNIT()
NAMED_UNIT(*)
SI_UNIT(.CENTI.,.METRE.)
);
#10269=(
NAMED_UNIT(*)
PLANE_ANGLE_UNIT()
SI_UNIT($,.RADIAN.)
);
#10270=(
NAMED_UNIT(*)
SI_UNIT($,.STERADIAN.)
SOLID_ANGLE_UNIT()
);
#10284=SHAPE_DEFINITION_REPRESENTATION(#10308,#10367);
#10308=PRODUCT_DEFINITION_SHAPE('',$,#10392);
#10367=SHAPE_REPRESENTATION('',(#5377),#10255);
#10378=PRODUCT_DEFINITION_CONTEXT('part definition',#10452,'design');
#10392=PRODUCT_DEFINITION('Control spring','Control spring',
#10416,#10378);
#10416=PRODUCT_DEFINITION_FORMATION('',$,#10467);
#10452=APPLICATION_CONTEXT(
'Core Data for Automotive Mechanical Design Process');
#10453=PRODUCT_CONTEXT('part definition',#10452,'mechanical');
#10467=PRODUCT('Control spring','Control spring',
'Control spring',(#10453));
#10541=COLOUR_RGB('Grey',0.48,0.52,0.57);
#10542=FILL_AREA_STYLE_COLOUR('',#10541);
#10543=FILL_AREA_STYLE('',(#10542));
#10544=SURFACE_STYLE_FILL_AREA(#10543);
#10545=SURFACE_SIDE_STYLE('',(#10544));
#10546=SURFACE_STYLE_USAGE(.BOTH.,#10545);
#10547=PRESENTATION_STYLE_ASSIGNMENT((#10546));
ENDSEC;
END-ISO-10303-21;
